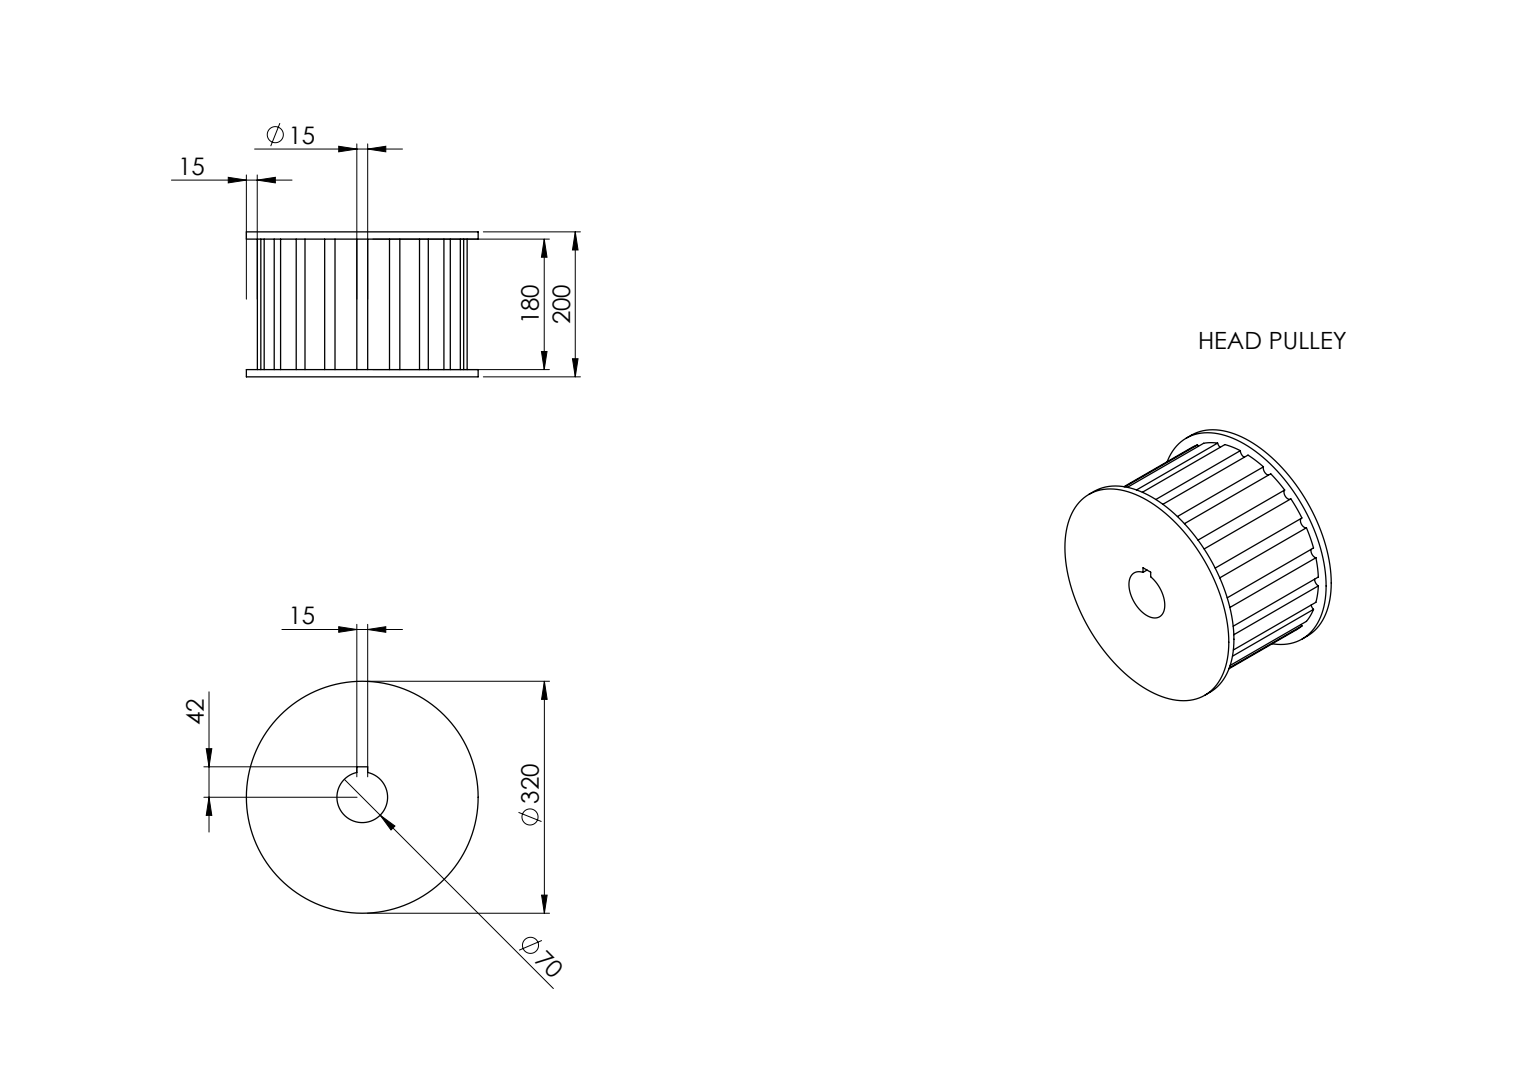
ISO-10303-21;
HEADER;
FILE_DESCRIPTION (('STEP AP214'),
    '1' );
FILE_NAME ('head pulley.step',
    '2026-10-31T03:46:07',
    ( '' ),
    ( '' ),
    'SwSTEP 2.0',
    'SolidWorks 2026',
    '' );
FILE_SCHEMA (( 'AUTOMOTIVE_DESIGN' ));
ENDSEC;

DATA;
#2=AXIS2_PLACEMENT_3D ( 'NONE', #6782, #12036, #15971 ) ;
#22=EDGE_CURVE ( 'NONE', #12572, #17693, #16078, .T. ) ;
#63=ORIENTED_EDGE ( 'NONE', *, *, #22259, .T. ) ;
#78=LINE ( 'NONE', #5499, #566 ) ;
#89=ORIENTED_EDGE ( 'NONE', *, *, #1676, .F. ) ;
#114=ORIENTED_EDGE ( 'NONE', *, *, #423, .T. ) ;
#116=EDGE_CURVE ( 'NONE', #3375, #7169, #11833, .T. ) ;
#119=DIRECTION ( 'NONE',  ( 1.000000000000000000, 0.000000000000000000, 0.000000000000000000 ) ) ;
#121=ORIENTED_EDGE ( 'NONE', *, *, #12195, .F. ) ;
#134=CARTESIAN_POINT ( 'NONE',  ( -91.18044947428953151, 112.7436279071528702, 90.00000000000000000 ) ) ;
#155=DIRECTION ( 'NONE',  ( -0.000000000000000000, 0.000000000000000000, 1.000000000000000000 ) ) ;
#158=EDGE_LOOP ( 'NONE', ( #17391, #12843, #343, #3950 ) ) ;
#213=CIRCLE ( 'NONE', #14875, 160.0000000000000000 ) ;
#217=CARTESIAN_POINT ( 'NONE',  ( 0.000000000000000000, 0.000000000000000000, 90.00000000000000000 ) ) ;
#229=DIRECTION ( 'NONE',  ( 0.000000000000000000, 0.000000000000000000, 1.000000000000000000 ) ) ;
#235=AXIS2_PLACEMENT_3D ( 'NONE', #16320, #23663, #13576 ) ;
#236=AXIS2_PLACEMENT_3D ( 'NONE', #4373, #19210, #636 ) ;
#258=LINE ( 'NONE', #11397, #17366 ) ;
#261=AXIS2_PLACEMENT_3D ( 'NONE', #2873, #10278, #8330 ) ;
#285=PRESENTATION_STYLE_ASSIGNMENT (( #3537 ) ) ;
#294=AXIS2_PLACEMENT_3D ( 'NONE', #882, #5000, #6440 ) ;
#298=LINE ( 'NONE', #3551, #3445 ) ;
#329=DIRECTION ( 'NONE',  ( 1.000000000000000000, 0.000000000000000000, 0.000000000000000000 ) ) ;
#333=AXIS2_PLACEMENT_3D ( 'NONE', #11581, #4410, #11450 ) ;
#343=ORIENTED_EDGE ( 'NONE', *, *, #12074, .F. ) ;
#369=VECTOR ( 'NONE', #13127, 1000.000000000000000 ) ;
#383=CARTESIAN_POINT ( 'NONE',  ( -144.8060344827586050, -7.497491405672223941, -2.775557561562891351E-14 ) ) ;
#395=CARTESIAN_POINT ( 'NONE',  ( 51.87806360044629628, 135.4018704341563364, -90.00000000000000000 ) ) ;
#399=CIRCLE ( 'NONE', #7721, 7.499999999999996447 ) ;
#402=EDGE_LOOP ( 'NONE', ( #16572, #22684, #22058, #9340 ) ) ;
#417=AXIS2_PLACEMENT_3D ( 'NONE', #10094, #19108, #10454 ) ;
#423=EDGE_CURVE ( 'NONE', #23301, #11044, #12932, .T. ) ;
#427=ADVANCED_FACE ( 'NONE', ( #15825 ), #831, .F. ) ;
#440=DIRECTION ( 'NONE',  ( 1.000000000000000000, 0.000000000000000000, 0.000000000000000000 ) ) ;
#450=ORIENTED_EDGE ( 'NONE', *, *, #16095, .T. ) ;
#452=CARTESIAN_POINT ( 'NONE',  ( 0.000000000000000000, 0.000000000000000000, 90.00000000000000000 ) ) ;
#461=EDGE_LOOP ( 'NONE', ( #908, #4370, #8639, #3777 ) ) ;
#466=DIRECTION ( 'NONE',  ( 0.000000000000000000, 0.000000000000000000, 1.000000000000000000 ) ) ;
#467=DIRECTION ( 'NONE',  ( 0.9510565162951580831, -0.3090169943749334069, 0.000000000000000000 ) ) ;
#501=EDGE_LOOP ( 'NONE', ( #8871, #21661, #12574, #4452 ) ) ;
#517=DIRECTION ( 'NONE',  ( -0.000000000000000000, -0.000000000000000000, 1.000000000000000000 ) ) ;
#519=ORIENTED_EDGE ( 'NONE', *, *, #14734, .F. ) ;
#533=ORIENTED_EDGE ( 'NONE', *, *, #2318, .F. ) ;
#536=FACE_OUTER_BOUND ( 'NONE', #16343, .T. ) ;
#548=DIRECTION ( 'NONE',  ( -3.700743415417187942E-15, 1.000000000000000000, 0.000000000000000000 ) ) ;
#554=CARTESIAN_POINT ( 'NONE',  ( 0.000000000000000000, 0.000000000000000000, -90.00000000000000000 ) ) ;
#566=VECTOR ( 'NONE', #11218, 1000.000000000000000 ) ;
#569=AXIS2_PLACEMENT_3D ( 'NONE', #10338, #15656, #17679 ) ;
#595=VECTOR ( 'NONE', #12133, 1000.000000000000000 ) ;
#599=ORIENTED_EDGE ( 'NONE', *, *, #1215, .T. ) ;
#601=VECTOR ( 'NONE', #6636, 1000.000000000000000 ) ;
#636=DIRECTION ( 'NONE',  ( 1.000000000000000000, 0.000000000000000000, 0.000000000000000000 ) ) ;
#649=CYLINDRICAL_SURFACE ( 'NONE', #1566, 160.0000000000000000 ) ;
#666=DIRECTION ( 'NONE',  ( -0.000000000000000000, -0.000000000000000000, 1.000000000000000000 ) ) ;
#669=CARTESIAN_POINT ( 'NONE',  ( 0.000000000000000000, 0.000000000000000000, -90.00000000000000000 ) ) ;
#680=ORIENTED_EDGE ( 'NONE', *, *, #10475, .T. ) ;
#701=CARTESIAN_POINT ( 'NONE',  ( 0.000000000000000000, 0.000000000000000000, -90.00000000000000000 ) ) ;
#724=LINE ( 'NONE', #11387, #3443 ) ;
#764=CIRCLE ( 'NONE', #10431, 7.500000000000000888 ) ;
#766=VERTEX_POINT ( 'NONE', #23002 ) ;
#772=ORIENTED_EDGE ( 'NONE', *, *, #4782, .T. ) ;
#796=DIRECTION ( 'NONE',  ( 0.000000000000000000, 0.000000000000000000, 1.000000000000000000 ) ) ;
#807=DIRECTION ( 'NONE',  ( 0.000000000000000000, -0.000000000000000000, 1.000000000000000000 ) ) ;
#811=CARTESIAN_POINT ( 'NONE',  ( 160.0000000000000000, 1.959434878635765210E-14, 100.0000000000000000 ) ) ;
#821=LINE ( 'NONE', #19284, #1182 ) ;
#831=CYLINDRICAL_SURFACE ( 'NONE', #5609, 7.500000000000007105 ) ;
#835=EDGE_CURVE ( 'NONE', #2765, #10209, #1509, .T. ) ;
#856=CARTESIAN_POINT ( 'NONE',  ( 37.61698748598423947, 140.0355749532214702, -90.00000000000000000 ) ) ;
#857=ORIENTED_EDGE ( 'NONE', *, *, #7014, .T. ) ;
#880=VERTEX_POINT ( 'NONE', #13468 ) ;
#882=CARTESIAN_POINT ( 'NONE',  ( -44.80746418436648071, -137.9031948627975908, -90.00000000000000000 ) ) ;
#884=LINE ( 'NONE', #23340, #6165 ) ;
#895=VECTOR ( 'NONE', #10102, 1000.000000000000000 ) ;
#906=CYLINDRICAL_SURFACE ( 'NONE', #17761, 145.0000000000000284 ) ;
#908=ORIENTED_EDGE ( 'NONE', *, *, #12705, .F. ) ;
#909=DIRECTION ( 'NONE',  ( 0.000000000000000000, 0.000000000000000000, 1.000000000000000000 ) ) ;
#915=CIRCLE ( 'NONE', #6313, 7.500000000000001776 ) ;
#921=CARTESIAN_POINT ( 'NONE',  ( 7.497491405671719455, 144.8060344827586334, 90.00000000000000000 ) ) ;
#923=ORIENTED_EDGE ( 'NONE', *, *, #16478, .F. ) ;
#947=LINE ( 'NONE', #17750, #601 ) ;
#952=AXIS2_PLACEMENT_3D ( 'NONE', #10071, #9939, #18964 ) ;
#976=CARTESIAN_POINT ( 'NONE',  ( 0.000000000000000000, 0.000000000000000000, -90.00000000000000000 ) ) ;
#991=EDGE_CURVE ( 'NONE', #20344, #17672, #1333, .T. ) ;
#1001=FACE_OUTER_BOUND ( 'NONE', #4174, .T. ) ;
#1004=DIRECTION ( 'NONE',  ( 1.000000000000000000, 0.000000000000000000, 0.000000000000000000 ) ) ;
#1009=DIRECTION ( 'NONE',  ( 0.000000000000000000, 0.000000000000000000, 1.000000000000000000 ) ) ;
#1016=DIRECTION ( 'NONE',  ( -0.000000000000000000, -0.000000000000000000, 1.000000000000000000 ) ) ;
#1032=DIRECTION ( 'NONE',  ( -0.000000000000000000, -0.000000000000000000, 1.000000000000000000 ) ) ;
#1040=CARTESIAN_POINT ( 'NONE',  ( 0.000000000000000000, 0.000000000000000000, -90.00000000000000000 ) ) ;
#1047=DIRECTION ( 'NONE',  ( 1.000000000000000000, 0.000000000000000000, 0.000000000000000000 ) ) ;
#1053=CYLINDRICAL_SURFACE ( 'NONE', #6841, 145.0000000000000284 ) ;
#1067=CYLINDRICAL_SURFACE ( 'NONE', #22936, 145.0000000000000284 ) ;
#1083=VECTOR ( 'NONE', #9378, 1000.000000000000000 ) ;
#1085=ORIENTED_EDGE ( 'NONE', *, *, #2157, .T. ) ;
#1091=CARTESIAN_POINT ( 'NONE',  ( -44.80746418436748968, 137.9031948627972781, 90.00000000000000000 ) ) ;
#1131=VERTEX_POINT ( 'NONE', #6538 ) ;
#1141=CARTESIAN_POINT ( 'NONE',  ( 144.8060344827585482, 7.497491405673236464, -90.00000000000000000 ) ) ;
#1148=VECTOR ( 'NONE', #21385, 1000.000000000000000 ) ;
#1149=DIRECTION ( 'NONE',  ( -0.000000000000000000, -0.000000000000000000, 1.000000000000000000 ) ) ;
#1154=DIRECTION ( 'NONE',  ( 1.000000000000000000, 0.000000000000000000, 0.000000000000000000 ) ) ;
#1165=AXIS2_PLACEMENT_3D ( 'NONE', #13877, #15664, #1154 ) ;
#1182=VECTOR ( 'NONE', #15686, 1000.000000000000000 ) ;
#1215=EDGE_CURVE ( 'NONE', #10931, #3015, #16546, .T. ) ;
#1229=CARTESIAN_POINT ( 'NONE',  ( 117.3074641843682144, -85.22886158240748955, -90.00000000000000000 ) ) ;
#1243=ORIENTED_EDGE ( 'NONE', *, *, #1911, .T. ) ;
#1244=EDGE_CURVE ( 'NONE', #12407, #10771, #17975, .T. ) ;
#1251=ORIENTED_EDGE ( 'NONE', *, *, #2208, .F. ) ;
#1256=CARTESIAN_POINT ( 'NONE',  ( 0.000000000000000000, 0.000000000000000000, -90.00000000000000000 ) ) ;
#1259=FACE_OUTER_BOUND ( 'NONE', #10230, .T. ) ;
#1263=FACE_OUTER_BOUND ( 'NONE', #6850, .T. ) ;
#1267=CARTESIAN_POINT ( 'NONE',  ( 0.000000000000000000, 0.000000000000000000, -90.00000000000000000 ) ) ;
#1278=CARTESIAN_POINT ( 'NONE',  ( 0.000000000000000000, 0.000000000000000000, -90.00000000000000000 ) ) ;
#1295=VERTEX_POINT ( 'NONE', #11268 ) ;
#1300=ADVANCED_FACE ( 'NONE', ( #18575 ), #14405, .F. ) ;
#1307=EDGE_CURVE ( 'NONE', #12981, #9371, #16811, .T. ) ;
#1312=DIRECTION ( 'NONE',  ( 0.000000000000000000, 0.000000000000000000, 1.000000000000000000 ) ) ;
#1316=CARTESIAN_POINT ( 'NONE',  ( -91.18044947428876412, -112.7436279071535239, -90.00000000000000000 ) ) ;
#1317=CIRCLE ( 'NONE', #7476, 7.499999999999996447 ) ;
#1322=VERTEX_POINT ( 'NONE', #17268 ) ;
#1323=DIRECTION ( 'NONE',  ( -0.000000000000000000, -0.000000000000000000, 1.000000000000000000 ) ) ;
#1333=CIRCLE ( 'NONE', #952, 145.0000000000000284 ) ;
#1368=CARTESIAN_POINT ( 'NONE',  ( -44.80746418436648071, -137.9031948627975908, -90.00000000000000000 ) ) ;
#1389=DIRECTION ( 'NONE',  ( 0.5877852522924826850, -0.8090169943749405679, 0.000000000000000000 ) ) ;
#1402=ORIENTED_EDGE ( 'NONE', *, *, #2339, .F. ) ;
#1406=FACE_OUTER_BOUND ( 'NONE', #5182, .T. ) ;
#1444=AXIS2_PLACEMENT_3D ( 'NONE', #23645, #5648, #23539 ) ;
#1456=CIRCLE ( 'NONE', #13459, 160.0000000000000000 ) ;
#1462=CARTESIAN_POINT ( 'NONE',  ( 0.000000000000000000, 0.000000000000000000, 100.0000000000000000 ) ) ;
#1480=ORIENTED_EDGE ( 'NONE', *, *, #116, .F. ) ;
#1486=ORIENTED_EDGE ( 'NONE', *, *, #8980, .T. ) ;
#1492=PRODUCT_DEFINITION_SHAPE ( 'NONE', 'NONE',  #21557 ) ;
#1498=AXIS2_PLACEMENT_3D ( 'NONE', #10621, #14371, #12334 ) ;
#1509=LINE ( 'NONE', #3191, #4429 ) ;
#1513=CIRCLE ( 'NONE', #7691, 7.500000000000001776 ) ;
#1514=CARTESIAN_POINT ( 'NONE',  ( 85.22886158240706322, 117.3074641843685129, -90.00000000000000000 ) ) ;
#1518=CIRCLE ( 'NONE', #16954, 7.499999999999998224 ) ;
#1533=DIRECTION ( 'NONE',  ( 0.000000000000000000, 0.000000000000000000, 1.000000000000000000 ) ) ;
#1541=DIRECTION ( 'NONE',  ( 0.000000000000000000, -0.000000000000000000, 1.000000000000000000 ) ) ;
#1565=CIRCLE ( 'NONE', #6182, 7.500000000000000888 ) ;
#1566=AXIS2_PLACEMENT_3D ( 'NONE', #2201, #7778, #5721 ) ;
#1570=DIRECTION ( 'NONE',  ( 1.000000000000000000, 0.000000000000000000, 0.000000000000000000 ) ) ;
#1571=ORIENTED_EDGE ( 'NONE', *, *, #18407, .T. ) ;
#1577=FACE_OUTER_BOUND ( 'NONE', #7495, .T. ) ;
#1579=DIRECTION ( 'NONE',  ( -0.000000000000000000, -0.000000000000000000, -1.000000000000000000 ) ) ;
#1582=ORIENTED_EDGE ( 'NONE', *, *, #991, .T. ) ;
#1595=CARTESIAN_POINT ( 'NONE',  ( -137.9031948627971076, -44.80746418436799416, -90.00000000000000000 ) ) ;
#1604=CARTESIAN_POINT ( 'NONE',  ( 0.000000000000000000, 0.000000000000000000, 90.00000000000000000 ) ) ;
#1629=PLANE ( 'NONE',  #11213 ) ;
#1634=DIRECTION ( 'NONE',  ( 0.3090169943749589421, -0.9510565162951498674, 0.000000000000000000 ) ) ;
#1676=EDGE_CURVE ( 'NONE', #18305, #13461, #5588, .T. ) ;
#1696=DIRECTION ( 'NONE',  ( -0.000000000000000000, -0.000000000000000000, -1.000000000000000000 ) ) ;
#1737=DIRECTION ( 'NONE',  ( 0.000000000000000000, -0.000000000000000000, 1.000000000000000000 ) ) ;
#1741=CARTESIAN_POINT ( 'NONE',  ( 145.0000000000000284, 1.518794382396763073E-12, -90.00000000000000000 ) ) ;
#1747=DIRECTION ( 'NONE',  ( 0.000000000000000000, 0.000000000000000000, 1.000000000000000000 ) ) ;
#1762=EDGE_CURVE ( 'NONE', #13072, #14205, #10366, .T. ) ;
#1784=CARTESIAN_POINT ( 'NONE',  ( 0.000000000000000000, 0.000000000000000000, -90.00000000000000000 ) ) ;
#1791=DIRECTION ( 'NONE',  ( 0.000000000000000000, -0.000000000000000000, 1.000000000000000000 ) ) ;
#1794=AXIS2_PLACEMENT_3D ( 'NONE', #14987, #11136, #18938 ) ;
#1827=CARTESIAN_POINT ( 'NONE',  ( -135.4018704341557680, 51.87806360044768184, -2.775557561562891351E-14 ) ) ;
#1876=DIRECTION ( 'NONE',  ( 0.8090169943749468962, 0.5877852522924740253, 0.000000000000000000 ) ) ;
#1883=AXIS2_PLACEMENT_3D ( 'NONE', #17096, #15181, #18896 ) ;
#1892=CARTESIAN_POINT ( 'NONE',  ( -121.5574576620394112, -79.04925354955290118, 90.00000000000000000 ) ) ;
#1908=CARTESIAN_POINT ( 'NONE',  ( -137.9031948627974486, 44.80746418436699940, -90.00000000000000000 ) ) ;
#1910=CIRCLE ( 'NONE', #9647, 7.499999999999998224 ) ;
#1911=EDGE_CURVE ( 'NONE', #17693, #2497, #16893, .T. ) ;
#1951=EDGE_CURVE ( 'NONE', #20344, #18305, #14697, .T. ) ;
#1977=ADVANCED_FACE ( 'NONE', ( #5259 ), #11076, .F. ) ;
#1997=DIRECTION ( 'NONE',  ( 0.000000000000000000, 0.000000000000000000, 1.000000000000000000 ) ) ;
#2001=AXIS2_PLACEMENT_3D ( 'NONE', #14523, #21858, #3611 ) ;
#2013=CARTESIAN_POINT ( 'NONE',  ( -77.72886158240795851, -117.3074641843678876, 90.00000000000000000 ) ) ;
#2032=EDGE_CURVE ( 'NONE', #17746, #2765, #11464, .T. ) ;
#2033=EDGE_CURVE ( 'NONE', #11764, #2480, #23769, .T. ) ;
#2046=CYLINDRICAL_SURFACE ( 'NONE', #9224, 145.0000000000000284 ) ;
#2077=CARTESIAN_POINT ( 'NONE',  ( -160.0000000000000000, 0.000000000000000000, 100.0000000000000000 ) ) ;
#2080=CARTESIAN_POINT ( 'NONE',  ( 112.7436279071538792, -91.18044947428829516, 90.00000000000000000 ) ) ;
#2081=ORIENTED_EDGE ( 'NONE', *, *, #10315, .T. ) ;
#2083=( LENGTH_UNIT ( ) NAMED_UNIT ( * ) SI_UNIT ( .MILLI., .METRE. ) );
#2090=DIRECTION ( 'NONE',  ( 0.000000000000000000, 0.000000000000000000, -1.000000000000000000 ) ) ;
#2094=CARTESIAN_POINT ( 'NONE',  ( 135.4018704341550290, 51.87806360044960030, -2.775557561562891351E-14 ) ) ;
#2121=DIRECTION ( 'NONE',  ( 0.000000000000000000, 0.000000000000000000, 1.000000000000000000 ) ) ;
#2129=PLANE ( 'NONE',  #2515 ) ;
#2155=ORIENTED_EDGE ( 'NONE', *, *, #11016, .F. ) ;
#2157=EDGE_CURVE ( 'NONE', #11764, #22779, #3251, .T. ) ;
#2159=AXIS2_PLACEMENT_3D ( 'NONE', #16619, #18062, #16480 ) ;
#2164=DIRECTION ( 'NONE',  ( -0.8090169943749507819, 0.5877852522924686962, 0.000000000000000000 ) ) ;
#2165=DIRECTION ( 'NONE',  ( 1.000000000000000000, 0.000000000000000000, 0.000000000000000000 ) ) ;
#2185=ORIENTED_EDGE ( 'NONE', *, *, #4517, .F. ) ;
#2187=CYLINDRICAL_SURFACE ( 'NONE', #236, 7.500000000000007105 ) ;
#2191=PLANE ( 'NONE',  #14998 ) ;
#2201=CARTESIAN_POINT ( 'NONE',  ( 0.000000000000000000, 0.000000000000000000, 100.0000000000000000 ) ) ;
#2202=AXIS2_PLACEMENT_3D ( 'NONE', #14375, #18086, #9030 ) ;
#2208=EDGE_CURVE ( 'NONE', #17463, #13673, #4416, .T. ) ;
#2230=VECTOR ( 'NONE', #5125, 1000.000000000000000 ) ;
#2239=DIRECTION ( 'NONE',  ( 0.000000000000000000, 0.000000000000000000, 1.000000000000000000 ) ) ;
#2252=DIRECTION ( 'NONE',  ( 0.000000000000000000, 0.000000000000000000, 1.000000000000000000 ) ) ;
#2258=PLANE ( 'NONE',  #4571 ) ;
#2283=AXIS2_PLACEMENT_3D ( 'NONE', #6230, #5097, #15543 ) ;
#2285=CIRCLE ( 'NONE', #16192, 145.0000000000000284 ) ;
#2292=VECTOR ( 'NONE', #4806, 1000.000000000000000 ) ;
#2303=ORIENTED_EDGE ( 'NONE', *, *, #4569, .F. ) ;
#2314=FACE_OUTER_BOUND ( 'NONE', #10322, .T. ) ;
#2317=CYLINDRICAL_SURFACE ( 'NONE', #4211, 145.0000000000000284 ) ;
#2318=EDGE_CURVE ( 'NONE', #16501, #13664, #5742, .T. ) ;
#2320=VERTEX_POINT ( 'NONE', #10099 ) ;
#2339=EDGE_CURVE ( 'NONE', #6206, #13931, #4971, .T. ) ;
#2351=DIRECTION ( 'NONE',  ( -0.000000000000000000, 0.000000000000000000, 1.000000000000000000 ) ) ;
#2361=CARTESIAN_POINT ( 'NONE',  ( 160.0000000000000000, 1.959434878635765210E-14, 100.0000000000000000 ) ) ;
#2370=CARTESIAN_POINT ( 'NONE',  ( 0.000000000000000000, 0.000000000000000000, 90.00000000000000000 ) ) ;
#2376=EDGE_CURVE ( 'NONE', #18600, #18149, #23477, .T. ) ;
#2406=ORIENTED_EDGE ( 'NONE', *, *, #20105, .T. ) ;
#2441=DIRECTION ( 'NONE',  ( 1.000000000000000000, 0.000000000000000000, 0.000000000000000000 ) ) ;
#2459=ORIENTED_EDGE ( 'NONE', *, *, #4998, .T. ) ;
#2461=CARTESIAN_POINT ( 'NONE',  ( 140.0355749532213281, -37.61698748598472264, 90.00000000000000000 ) ) ;
#2475=DIRECTION ( 'NONE',  ( 0.000000000000000000, 0.000000000000000000, 1.000000000000000000 ) ) ;
#2480=VERTEX_POINT ( 'NONE', #5349 ) ;
#2483=LINE ( 'NONE', #20962, #9282 ) ;
#2497=VERTEX_POINT ( 'NONE', #8874 ) ;
#2509=ORIENTED_EDGE ( 'NONE', *, *, #11719, .T. ) ;
#2515=AXIS2_PLACEMENT_3D ( 'NONE', #3941, #7574, #9521 ) ;
#2575=EDGE_CURVE ( 'NONE', #3378, #2646, #3889, .T. ) ;
#2579=ORIENTED_EDGE ( 'NONE', *, *, #13734, .F. ) ;
#2601=EDGE_CURVE ( 'NONE', #1295, #18149, #20390, .T. ) ;
#2612=EDGE_LOOP ( 'NONE', ( #8421, #21186, #22709, #21255 ) ) ;
#2636=EDGE_CURVE ( 'NONE', #21483, #4937, #16940, .T. ) ;
#2644=LINE ( 'NONE', #6511, #4380 ) ;
#2645=ORIENTED_EDGE ( 'NONE', *, *, #6630, .T. ) ;
#2646=VERTEX_POINT ( 'NONE', #16812 ) ;
#2653=AXIS2_PLACEMENT_3D ( 'NONE', #18912, #22648, #19018 ) ;
#2663=ADVANCED_FACE ( 'NONE', ( #5831 ), #2317, .T. ) ;
#2667=CARTESIAN_POINT ( 'NONE',  ( -37.61698748598514896, -140.0355749532212428, -2.775557561562891351E-14 ) ) ;
#2670=AXIS2_PLACEMENT_3D ( 'NONE', #17531, #19703, #21287 ) ;
#2676=CARTESIAN_POINT ( 'NONE',  ( -51.87806360044817922, 135.4018704341556258, -2.775557561562891351E-14 ) ) ;
#2684=ORIENTED_EDGE ( 'NONE', *, *, #6466, .F. ) ;
#2710=DIRECTION ( 'NONE',  ( 0.3090169943749441761, 0.9510565162951546414, 0.000000000000000000 ) ) ;
#2716=LINE ( 'NONE', #21061, #895 ) ;
#2720=ORIENTED_EDGE ( 'NONE', *, *, #16990, .F. ) ;
#2745=DIRECTION ( 'NONE',  ( 1.000000000000000000, 0.000000000000000000, 0.000000000000000000 ) ) ;
#2747=DIRECTION ( 'NONE',  ( -0.000000000000000000, 0.000000000000000000, 1.000000000000000000 ) ) ;
#2760=EDGE_LOOP ( 'NONE', ( #18334, #15913 ) ) ;
#2765=VERTEX_POINT ( 'NONE', #15377 ) ;
#2777=EDGE_CURVE ( 'NONE', #9321, #21395, #16651, .T. ) ;
#2803=LINE ( 'NONE', #15632, #15852 ) ;
#2826=CARTESIAN_POINT ( 'NONE',  ( -44.80746418436648071, -137.9031948627975908, 90.00000000000000000 ) ) ;
#2829=DIRECTION ( 'NONE',  ( 0.000000000000000000, 0.000000000000000000, 1.000000000000000000 ) ) ;
#2831=DIRECTION ( 'NONE',  ( 1.000000000000000000, 0.000000000000000000, 0.000000000000000000 ) ) ;
#2844=ORIENTED_EDGE ( 'NONE', *, *, #19085, .F. ) ;
#2852=CARTESIAN_POINT ( 'NONE',  ( -112.7436279071531828, 91.18044947428913360, -90.00000000000000000 ) ) ;
#2854=AXIS2_PLACEMENT_3D ( 'NONE', #16273, #21451, #1634 ) ;
#2873=CARTESIAN_POINT ( 'NONE',  ( 0.000000000000000000, 0.000000000000000000, -90.00000000000000000 ) ) ;
#2874=AXIS2_PLACEMENT_3D ( 'NONE', #20053, #18347, #8961 ) ;
#2877=CARTESIAN_POINT ( 'NONE',  ( 79.04925354955072692, 121.5574576620408322, 90.00000000000000000 ) ) ;
#2884=CIRCLE ( 'NONE', #9085, 145.0000000000000284 ) ;
#2912=CIRCLE ( 'NONE', #18734, 145.0000000000000284 ) ;
#2914=DIRECTION ( 'NONE',  ( 0.000000000000000000, 0.000000000000000000, -1.000000000000000000 ) ) ;
#2919=ORIENTED_EDGE ( 'NONE', *, *, #13068, .T. ) ;
#2944=EDGE_CURVE ( 'NONE', #15856, #9608, #22362, .T. ) ;
#2947=ORIENTED_EDGE ( 'NONE', *, *, #20986, .F. ) ;
#2957=CARTESIAN_POINT ( 'NONE',  ( 85.22886158240964960, -117.3074641843666370, 90.00000000000000000 ) ) ;
#2990=DIRECTION ( 'NONE',  ( 1.000000000000000000, 0.000000000000000000, 0.000000000000000000 ) ) ;
#3015=VERTEX_POINT ( 'NONE', #10497 ) ;
#3031=EDGE_CURVE ( 'NONE', #21305, #6640, #16542, .T. ) ;
#3070=CARTESIAN_POINT ( 'NONE',  ( -7.497491405671719455, 144.8060344827586334, -2.775557561562891351E-14 ) ) ;
#3075=EDGE_LOOP ( 'NONE', ( #16565, #17357, #19371, #4735, #9836, #18694 ) ) ;
#3108=AXIS2_PLACEMENT_3D ( 'NONE', #16381, #1747, #18295 ) ;
#3110=VERTEX_POINT ( 'NONE', #6364 ) ;
#3130=CARTESIAN_POINT ( 'NONE',  ( 112.7436279071518612, 91.18044947429076785, 90.00000000000000000 ) ) ;
#3142=VERTEX_POINT ( 'NONE', #921 ) ;
#3152=DIRECTION ( 'NONE',  ( 1.000000000000000000, 0.000000000000000000, 0.000000000000000000 ) ) ;
#3182=CARTESIAN_POINT ( 'NONE',  ( -112.7436279071525433, -91.18044947428992941, 90.00000000000000000 ) ) ;
#3185=ORIENTED_EDGE ( 'NONE', *, *, #10970, .T. ) ;
#3187=ORIENTED_EDGE ( 'NONE', *, *, #3737, .F. ) ;
#3191=CARTESIAN_POINT ( 'NONE',  ( -37.61698748598617925, 140.0355749532209870, -2.775557561562891351E-14 ) ) ;
#3207=DIRECTION ( 'NONE',  ( -0.000000000000000000, -0.000000000000000000, 1.000000000000000000 ) ) ;
#3239=DIRECTION ( 'NONE',  ( 0.000000000000000000, 0.000000000000000000, 1.000000000000000000 ) ) ;
#3241=EDGE_CURVE ( 'NONE', #5473, #13502, #5147, .T. ) ;
#3251=CIRCLE ( 'NONE', #22915, 7.500000000000004441 ) ;
#3258=CIRCLE ( 'NONE', #9468, 160.0000000000000000 ) ;
#3267=DIRECTION ( 'NONE',  ( 0.000000000000000000, -0.000000000000000000, 1.000000000000000000 ) ) ;
#3291=AXIS2_PLACEMENT_3D ( 'NONE', #1256, #10212, #10333 ) ;
#3299=CARTESIAN_POINT ( 'NONE',  ( -79.04925354955163641, -121.5574576620402496, -90.00000000000000000 ) ) ;
#3305=EDGE_CURVE ( 'NONE', #12407, #18161, #19576, .T. ) ;
#3326=DIRECTION ( 'NONE',  ( 1.000000000000000000, 0.000000000000000000, 0.000000000000000000 ) ) ;
#3331=ADVANCED_FACE ( 'NONE', ( #6798 ), #8503, .F. ) ;
#3350=VECTOR ( 'NONE', #14502, 1000.000000000000000 ) ;
#3360=CARTESIAN_POINT ( 'NONE',  ( 0.000000000000000000, 0.000000000000000000, 100.0000000000000000 ) ) ;
#3370=CARTESIAN_POINT ( 'NONE',  ( 85.22886158240964960, -117.3074641843666370, -90.00000000000000000 ) ) ;
#3375=VERTEX_POINT ( 'NONE', #13973 ) ;
#3378=VERTEX_POINT ( 'NONE', #12156 ) ;
#3380=VECTOR ( 'NONE', #3868, 1000.000000000000000 ) ;
#3385=AXIS2_PLACEMENT_3D ( 'NONE', #22286, #16863, #17233 ) ;
#3401=VECTOR ( 'NONE', #9352, 1000.000000000000000 ) ;
#3407=CARTESIAN_POINT ( 'NONE',  ( 0.000000000000000000, 0.000000000000000000, -90.00000000000000000 ) ) ;
#3421=VECTOR ( 'NONE', #4763, 1000.000000000000000 ) ;
#3429=ORIENTED_EDGE ( 'NONE', *, *, #21555, .F. ) ;
#3443=VECTOR ( 'NONE', #13694, 1000.000000000000000 ) ;
#3445=VECTOR ( 'NONE', #1737, 1000.000000000000000 ) ;
#3446=VECTOR ( 'NONE', #13913, 1000.000000000000000 ) ;
#3471=CARTESIAN_POINT ( 'NONE',  ( 0.000000000000000000, 0.000000000000000000, -100.0000000000000000 ) ) ;
#3475=VECTOR ( 'NONE', #2914, 1000.000000000000000 ) ;
#3483=CARTESIAN_POINT ( 'NONE',  ( -85.22886158240879695, 117.3074641843673049, -90.00000000000000000 ) ) ;
#3489=AXIS2_PLACEMENT_3D ( 'NONE', #13729, #22848, #11795 ) ;
#3497=DIRECTION ( 'NONE',  ( 1.000000000000000000, 0.000000000000000000, 0.000000000000000000 ) ) ;
#3517=ORIENTED_EDGE ( 'NONE', *, *, #16077, .T. ) ;
#3524=ORIENTED_EDGE ( 'NONE', *, *, #13067, .F. ) ;
#3537=SURFACE_STYLE_USAGE ( .BOTH. , #16715 ) ;
#3543=CARTESIAN_POINT ( 'NONE',  ( 0.000000000000000000, 0.000000000000000000, -90.00000000000000000 ) ) ;
#3545=EDGE_CURVE ( 'NONE', #7634, #10526, #9256, .T. ) ;
#3551=CARTESIAN_POINT ( 'NONE',  ( -79.04925354955163641, -121.5574576620402496, -2.775557561562891351E-14 ) ) ;
#3587=ORIENTED_EDGE ( 'NONE', *, *, #6215, .T. ) ;
#3611=DIRECTION ( 'NONE',  ( 0.3090169943749441761, 0.9510565162951546414, 0.000000000000000000 ) ) ;
#3633=EDGE_CURVE ( 'NONE', #13320, #22438, #298, .T. ) ;
#3650=DIRECTION ( 'NONE',  ( 1.000000000000000000, 0.000000000000000000, 0.000000000000000000 ) ) ;
#3670=CARTESIAN_POINT ( 'NONE',  ( 112.7436279071538792, -91.18044947428829516, -90.00000000000000000 ) ) ;
#3685=CARTESIAN_POINT ( 'NONE',  ( 0.000000000000000000, 0.000000000000000000, 90.00000000000000000 ) ) ;
#3693=VERTEX_POINT ( 'NONE', #15407 ) ;
#3694=EDGE_CURVE ( 'NONE', #12407, #19135, #4150, .T. ) ;
#3723=DIRECTION ( 'NONE',  ( 0.000000000000000000, 0.000000000000000000, 1.000000000000000000 ) ) ;
#3735=LINE ( 'NONE', #16913, #3380 ) ;
#3737=EDGE_CURVE ( 'NONE', #19135, #13502, #884, .T. ) ;
#3755=CIRCLE ( 'NONE', #17284, 7.499999999999998224 ) ;
#3769=DIRECTION ( 'NONE',  ( 1.000000000000000000, 0.000000000000000000, 0.000000000000000000 ) ) ;
#3777=ORIENTED_EDGE ( 'NONE', *, *, #8405, .F. ) ;
#3796=CARTESIAN_POINT ( 'NONE',  ( 135.4018704341561374, -51.87806360044677945, -2.775557561562891351E-14 ) ) ;
#3828=EDGE_LOOP ( 'NONE', ( #13650, #12892, #17242, #8630 ) ) ;
#3849=EDGE_CURVE ( 'NONE', #9726, #1322, #23504, .T. ) ;
#3859=AXIS2_PLACEMENT_3D ( 'NONE', #14257, #5168, #17735 ) ;
#3868=DIRECTION ( 'NONE',  ( 0.000000000000000000, -0.000000000000000000, 1.000000000000000000 ) ) ;
#3877=ORIENTED_EDGE ( 'NONE', *, *, #18176, .T. ) ;
#3883=EDGE_CURVE ( 'NONE', #22438, #17622, #9242, .T. ) ;
#3889=LINE ( 'NONE', #1827, #19244 ) ;
#3897=LINE ( 'NONE', #20550, #18071 ) ;
#3906=DIRECTION ( 'NONE',  ( 1.000000000000000000, 0.000000000000000000, 0.000000000000000000 ) ) ;
#3912=DIRECTION ( 'NONE',  ( 0.000000000000000000, 0.000000000000000000, 1.000000000000000000 ) ) ;
#3941=CARTESIAN_POINT ( 'NONE',  ( 7.499999999999999112, 0.000000000000000000, -100.0000000000000000 ) ) ;
#3950=ORIENTED_EDGE ( 'NONE', *, *, #21410, .F. ) ;
#3958=EDGE_LOOP ( 'NONE', ( #23510, #8785, #8693, #9032 ) ) ;
#3974=CARTESIAN_POINT ( 'NONE',  ( -85.22886158240795851, -117.3074641843678876, -90.00000000000000000 ) ) ;
#3976=DIRECTION ( 'NONE',  ( -0.000000000000000000, -0.000000000000000000, 1.000000000000000000 ) ) ;
#3988=AXIS2_PLACEMENT_3D ( 'NONE', #15544, #17350, #4660 ) ;
#4000=LINE ( 'NONE', #13608, #10803 ) ;
#4001=FACE_OUTER_BOUND ( 'NONE', #12359, .T. ) ;
#4031=CARTESIAN_POINT ( 'NONE',  ( -77.72886158240878274, 117.3074641843673049, -90.00000000000000000 ) ) ;
#4048=CYLINDRICAL_SURFACE ( 'NONE', #2653, 160.0000000000000000 ) ;
#4075=ADVANCED_FACE ( 'NONE', ( #8134 ), #22476, .F. ) ;
#4109=EDGE_CURVE ( 'NONE', #11121, #15263, #8595, .T. ) ;
#4114=VERTEX_POINT ( 'NONE', #14301 ) ;
#4115=ADVANCED_FACE ( 'NONE', ( #8484 ), #21150, .F. ) ;
#4119=ORIENTED_EDGE ( 'NONE', *, *, #15493, .F. ) ;
#4126=DIRECTION ( 'NONE',  ( -0.000000000000000000, -0.000000000000000000, 1.000000000000000000 ) ) ;
#4150=LINE ( 'NONE', #22390, #4613 ) ;
#4165=DIRECTION ( 'NONE',  ( -0.000000000000000000, -0.000000000000000000, 1.000000000000000000 ) ) ;
#4166=AXIS2_PLACEMENT_3D ( 'NONE', #1514, #18396, #9255 ) ;
#4174=EDGE_LOOP ( 'NONE', ( #13858, #6378, #10101, #1243 ) ) ;
#4177=DIRECTION ( 'NONE',  ( 0.000000000000000000, 0.000000000000000000, 1.000000000000000000 ) ) ;
#4185=FACE_OUTER_BOUND ( 'NONE', #13720, .T. ) ;
#4197=CARTESIAN_POINT ( 'NONE',  ( -35.00000000000000711, 4.286263797015737285E-15, -100.0000000000000000 ) ) ;
#4204=CIRCLE ( 'NONE', #18115, 145.0000000000000284 ) ;
#4211=AXIS2_PLACEMENT_3D ( 'NONE', #11177, #18722, #15143 ) ;
#4229=CARTESIAN_POINT ( 'NONE',  ( 160.0000000000000000, 1.959434878635765210E-14, -90.00000000000000000 ) ) ;
#4248=ORIENTED_EDGE ( 'NONE', *, *, #3545, .F. ) ;
#4258=DIRECTION ( 'NONE',  ( 1.000000000000000000, 0.000000000000000000, 0.000000000000000000 ) ) ;
#4260=ORIENTED_EDGE ( 'NONE', *, *, #22259, .F. ) ;
#4262=ADVANCED_FACE ( 'NONE', ( #10789 ), #16213, .F. ) ;
#4268=VERTEX_POINT ( 'NONE', #16553 ) ;
#4275=DIRECTION ( 'NONE',  ( -0.000000000000000000, -0.000000000000000000, 1.000000000000000000 ) ) ;
#4280=CARTESIAN_POINT ( 'NONE',  ( 0.000000000000000000, 145.0000000000000284, -90.00000000000000000 ) ) ;
#4287=ORIENTED_EDGE ( 'NONE', *, *, #12558, .F. ) ;
#4290=ORIENTED_EDGE ( 'NONE', *, *, #2376, .T. ) ;
#4310=LINE ( 'NONE', #6244, #6893 ) ;
#4327=DIRECTION ( 'NONE',  ( 0.000000000000000000, 0.000000000000000000, 1.000000000000000000 ) ) ;
#4338=DIRECTION ( 'NONE',  ( -0.000000000000000000, -0.000000000000000000, 1.000000000000000000 ) ) ;
#4365=DIRECTION ( 'NONE',  ( -0.000000000000000000, -0.000000000000000000, -1.000000000000000000 ) ) ;
#4370=ORIENTED_EDGE ( 'NONE', *, *, #8154, .T. ) ;
#4373=CARTESIAN_POINT ( 'NONE',  ( -145.0000000000000284, -5.062647941322544249E-13, -90.00000000000000000 ) ) ;
#4380=VECTOR ( 'NONE', #17614, 1000.000000000000000 ) ;
#4389=CARTESIAN_POINT ( 'NONE',  ( 35.00000000000000711, 0.000000000000000000, -100.0000000000000000 ) ) ;
#4404=ORIENTED_EDGE ( 'NONE', *, *, #6169, .T. ) ;
#4410=DIRECTION ( 'NONE',  ( 0.000000000000000000, 0.000000000000000000, 1.000000000000000000 ) ) ;
#4416=CIRCLE ( 'NONE', #13715, 7.500000000000000000 ) ;
#4427=AXIS2_PLACEMENT_3D ( 'NONE', #17887, #21386, #11899 ) ;
#4429=VECTOR ( 'NONE', #12549, 1000.000000000000000 ) ;
#4432=EDGE_CURVE ( 'NONE', #10931, #5086, #3258, .T. ) ;
#4452=ORIENTED_EDGE ( 'NONE', *, *, #13396, .F. ) ;
#4486=VECTOR ( 'NONE', #2090, 1000.000000000000000 ) ;
#4488=CARTESIAN_POINT ( 'NONE',  ( 0.000000000000000000, 0.000000000000000000, 90.00000000000000000 ) ) ;
#4489=ORIENTED_EDGE ( 'NONE', *, *, #17444, .T. ) ;
#4490=EDGE_CURVE ( 'NONE', #766, #5818, #11806, .T. ) ;
#4514=DIRECTION ( 'NONE',  ( -0.000000000000000000, 1.000000000000000000, 0.000000000000000000 ) ) ;
#4516=VERTEX_POINT ( 'NONE', #12114 ) ;
#4517=EDGE_CURVE ( 'NONE', #22779, #17746, #947, .T. ) ;
#4521=CYLINDRICAL_SURFACE ( 'NONE', #15666, 7.500000000000007105 ) ;
#4522=ORIENTED_EDGE ( 'NONE', *, *, #8740, .T. ) ;
#4527=DIRECTION ( 'NONE',  ( -0.9510565162951557516, 0.3090169943749406234, 0.000000000000000000 ) ) ;
#4535=CIRCLE ( 'NONE', #294, 7.500000000000000000 ) ;
#4537=AXIS2_PLACEMENT_3D ( 'NONE', #1462, #1696, #8851 ) ;
#4539=ORIENTED_EDGE ( 'NONE', *, *, #13068, .F. ) ;
#4548=ADVANCED_FACE ( 'NONE', ( #12357 ), #1067, .T. ) ;
#4558=CIRCLE ( 'NONE', #3385, 7.500000000000002665 ) ;
#4563=CARTESIAN_POINT ( 'NONE',  ( 7.499999999999999112, 0.000000000000000000, -100.0000000000000000 ) ) ;
#4567=CARTESIAN_POINT ( 'NONE',  ( -130.4031948627971076, -44.80746418436799416, -90.00000000000000000 ) ) ;
#4569=EDGE_CURVE ( 'NONE', #21305, #13461, #20628, .T. ) ;
#4571=AXIS2_PLACEMENT_3D ( 'NONE', #1784, #229, #9662 ) ;
#4613=VECTOR ( 'NONE', #4514, 1000.000000000000000 ) ;
#4631=ORIENTED_EDGE ( 'NONE', *, *, #1244, .T. ) ;
#4637=CARTESIAN_POINT ( 'NONE',  ( -121.5574576620393970, -79.04925354955290118, -2.775557561562891351E-14 ) ) ;
#4660=DIRECTION ( 'NONE',  ( 1.000000000000000000, 0.000000000000000000, 0.000000000000000000 ) ) ;
#4685=CARTESIAN_POINT ( 'NONE',  ( -140.0355749532211007, 37.61698748598567477, 90.00000000000000000 ) ) ;
#4735=ORIENTED_EDGE ( 'NONE', *, *, #1244, .F. ) ;
#4752=CARTESIAN_POINT ( 'NONE',  ( -137.9031948627971076, -44.80746418436799416, 90.00000000000000000 ) ) ;
#4754=VERTEX_POINT ( 'NONE', #9611 ) ;
#4759=EDGE_CURVE ( 'NONE', #5473, #13664, #21188, .T. ) ;
#4763=DIRECTION ( 'NONE',  ( 1.000000000000000000, 0.000000000000000000, 0.000000000000000000 ) ) ;
#4782=EDGE_CURVE ( 'NONE', #6740, #13908, #2884, .T. ) ;
#4786=CARTESIAN_POINT ( 'NONE',  ( -7.499999999999999112, 0.000000000000000000, -100.0000000000000000 ) ) ;
#4790=ADVANCED_FACE ( 'NONE', ( #17337 ), #4521, .F. ) ;
#4806=DIRECTION ( 'NONE',  ( -0.000000000000000000, 0.000000000000000000, -1.000000000000000000 ) ) ;
#4807=ORIENTED_EDGE ( 'NONE', *, *, #18145, .F. ) ;
#4842=ORIENTED_EDGE ( 'NONE', *, *, #21593, .F. ) ;
#4875=DIRECTION ( 'NONE',  ( 0.000000000000000000, 0.000000000000000000, 1.000000000000000000 ) ) ;
#4884=DIRECTION ( 'NONE',  ( 0.000000000000000000, -0.000000000000000000, 1.000000000000000000 ) ) ;
#4918=DIRECTION ( 'NONE',  ( 0.000000000000000000, 0.000000000000000000, 1.000000000000000000 ) ) ;
#4923=DIRECTION ( 'NONE',  ( -0.000000000000000000, 1.000000000000000000, 0.000000000000000000 ) ) ;
#4924=ORIENTED_EDGE ( 'NONE', *, *, #8154, .F. ) ;
#4927=DIRECTION ( 'NONE',  ( -3.700743415417187942E-15, 1.000000000000000000, 0.000000000000000000 ) ) ;
#4933=AXIS2_PLACEMENT_3D ( 'NONE', #14102, #10595, #3650 ) ;
#4937=VERTEX_POINT ( 'NONE', #12288 ) ;
#4943=DIRECTION ( 'NONE',  ( -0.8090169943749507819, 0.5877852522924686962, 0.000000000000000000 ) ) ;
#4959=AXIS2_PLACEMENT_3D ( 'NONE', #15194, #2121, #22885 ) ;
#4971=CIRCLE ( 'NONE', #17321, 7.500000000000002665 ) ;
#4977=DIRECTION ( 'NONE',  ( 0.000000000000000000, 0.000000000000000000, 1.000000000000000000 ) ) ;
#4987=FACE_OUTER_BOUND ( 'NONE', #19860, .T. ) ;
#4997=ORIENTED_EDGE ( 'NONE', *, *, #13396, .T. ) ;
#4998=EDGE_CURVE ( 'NONE', #5086, #10931, #9102, .T. ) ;
#5000=DIRECTION ( 'NONE',  ( 0.000000000000000000, 0.000000000000000000, 1.000000000000000000 ) ) ;
#5023=DIRECTION ( 'NONE',  ( -0.9510565162951557516, 0.3090169943749406234, 0.000000000000000000 ) ) ;
#5027=DIRECTION ( 'NONE',  ( -0.000000000000000000, -0.000000000000000000, 1.000000000000000000 ) ) ;
#5034=CIRCLE ( 'NONE', #16228, 7.500000000000002665 ) ;
#5050=EDGE_CURVE ( 'NONE', #17172, #5473, #20265, .T. ) ;
#5086=VERTEX_POINT ( 'NONE', #20086 ) ;
#5097=DIRECTION ( 'NONE',  ( 0.000000000000000000, 0.000000000000000000, 1.000000000000000000 ) ) ;
#5103=AXIS2_PLACEMENT_3D ( 'NONE', #3974, #11388, #2164 ) ;
#5125=DIRECTION ( 'NONE',  ( -0.000000000000000000, -0.000000000000000000, 1.000000000000000000 ) ) ;
#5128=CARTESIAN_POINT ( 'NONE',  ( 137.9031948627977044, -44.80746418436605438, 90.00000000000000000 ) ) ;
#5147=LINE ( 'NONE', #19985, #7654 ) ;
#5148=AXIS2_PLACEMENT_3D ( 'NONE', #7883, #6305, #19333 ) ;
#5159=EDGE_LOOP ( 'NONE', ( #22553, #4290, #12848, #10050 ) ) ;
#5168=DIRECTION ( 'NONE',  ( 0.000000000000000000, 0.000000000000000000, 1.000000000000000000 ) ) ;
#5181=ORIENTED_EDGE ( 'NONE', *, *, #22626, .F. ) ;
#5182=EDGE_LOOP ( 'NONE', ( #12131, #9938, #6429, #12883 ) ) ;
#5194=ADVANCED_FACE ( 'NONE', ( #7157 ), #11532, .F. ) ;
#5214=ADVANCED_FACE ( 'NONE', ( #17423 ), #2187, .F. ) ;
#5228=CIRCLE ( 'NONE', #18315, 160.0000000000000000 ) ;
#5242=CARTESIAN_POINT ( 'NONE',  ( -7.499999999999999112, 34.18698582794336716, 100.0000000000000000 ) ) ;
#5244=DIRECTION ( 'NONE',  ( 0.000000000000000000, 0.000000000000000000, -1.000000000000000000 ) ) ;
#5259=FACE_OUTER_BOUND ( 'NONE', #23081, .T. ) ;
#5263=CARTESIAN_POINT ( 'NONE',  ( 0.000000000000000000, 0.000000000000000000, -90.00000000000000000 ) ) ;
#5276=ORIENTED_EDGE ( 'NONE', *, *, #9577, .F. ) ;
#5289=DIRECTION ( 'NONE',  ( -0.5877852522924643663, -0.8090169943749537795, 0.000000000000000000 ) ) ;
#5293=ORIENTED_EDGE ( 'NONE', *, *, #22472, .T. ) ;
#5296=VECTOR ( 'NONE', #22077, 1000.000000000000000 ) ;
#5336=ORIENTED_EDGE ( 'NONE', *, *, #9820, .F. ) ;
#5347=CIRCLE ( 'NONE', #23073, 7.500000000000002665 ) ;
#5349=CARTESIAN_POINT ( 'NONE',  ( -79.04925354955248906, 121.5574576620396812, -90.00000000000000000 ) ) ;
#5357=CARTESIAN_POINT ( 'NONE',  ( -160.0000000000000000, 0.000000000000000000, 100.0000000000000000 ) ) ;
#5368=CIRCLE ( 'NONE', #18842, 145.0000000000000284 ) ;
#5399=DIRECTION ( 'NONE',  ( 1.000000000000000000, 0.000000000000000000, 0.000000000000000000 ) ) ;
#5430=AXIS2_PLACEMENT_3D ( 'NONE', #23089, #8257, #19455 ) ;
#5462=ADVANCED_FACE ( 'NONE', ( #8597 ), #23431, .T. ) ;
#5473=VERTEX_POINT ( 'NONE', #7242 ) ;
#5481=ORIENTED_EDGE ( 'NONE', *, *, #2601, .F. ) ;
#5489=CIRCLE ( 'NONE', #2001, 7.500000000000002665 ) ;
#5499=CARTESIAN_POINT ( 'NONE',  ( 51.87806360044628917, 135.4018704341563080, -2.775557561562891351E-14 ) ) ;
#5515=DIRECTION ( 'NONE',  ( -0.000000000000000000, -0.000000000000000000, 1.000000000000000000 ) ) ;
#5520=AXIS2_PLACEMENT_3D ( 'NONE', #15763, #8386, #11695 ) ;
#5554=AXIS2_PLACEMENT_3D ( 'NONE', #2826, #796, #4527 ) ;
#5564=CARTESIAN_POINT ( 'NONE',  ( 0.000000000000000000, 0.000000000000000000, -90.00000000000000000 ) ) ;
#5569=ORIENTED_EDGE ( 'NONE', *, *, #6770, .F. ) ;
#5575=EDGE_LOOP ( 'NONE', ( #23599, #7158, #7140, #20153 ) ) ;
#5586=ORIENTED_EDGE ( 'NONE', *, *, #21071, .F. ) ;
#5588=CIRCLE ( 'NONE', #19073, 7.500000000000002665 ) ;
#5609=AXIS2_PLACEMENT_3D ( 'NONE', #6745, #8320, #13920 ) ;
#5648=DIRECTION ( 'NONE',  ( -0.000000000000000000, -0.000000000000000000, 1.000000000000000000 ) ) ;
#5651=VERTEX_POINT ( 'NONE', #13692 ) ;
#5656=FACE_OUTER_BOUND ( 'NONE', #17417, .T. ) ;
#5701=DIRECTION ( 'NONE',  ( -3.700743415417187942E-15, 1.000000000000000000, 0.000000000000000000 ) ) ;
#5721=DIRECTION ( 'NONE',  ( -1.000000000000000000, 0.000000000000000000, 0.000000000000000000 ) ) ;
#5742=CIRCLE ( 'NONE', #9221, 35.00000000000000711 ) ;
#5758=DIRECTION ( 'NONE',  ( -0.000000000000000000, -0.000000000000000000, 1.000000000000000000 ) ) ;
#5759=ORIENTED_EDGE ( 'NONE', *, *, #14624, .T. ) ;
#5762=CYLINDRICAL_SURFACE ( 'NONE', #8124, 35.00000000000000711 ) ;
#5790=FACE_BOUND ( 'NONE', #22978, .T. ) ;
#5797=FACE_OUTER_BOUND ( 'NONE', #19410, .T. ) ;
#5811=ORIENTED_EDGE ( 'NONE', *, *, #23434, .F. ) ;
#5818=VERTEX_POINT ( 'NONE', #1316 ) ;
#5827=ORIENTED_EDGE ( 'NONE', *, *, #3694, .F. ) ;
#5828=DIRECTION ( 'NONE',  ( 0.000000000000000000, 0.000000000000000000, 1.000000000000000000 ) ) ;
#5831=FACE_OUTER_BOUND ( 'NONE', #15927, .T. ) ;
#5841=ORIENTED_EDGE ( 'NONE', *, *, #8556, .T. ) ;
#5874=DIRECTION ( 'NONE',  ( 0.000000000000000000, 0.000000000000000000, 1.000000000000000000 ) ) ;
#5910=ORIENTED_EDGE ( 'NONE', *, *, #11723, .T. ) ;
#5917=EDGE_CURVE ( 'NONE', #10526, #11121, #16600, .T. ) ;
#5924=EDGE_CURVE ( 'NONE', #10981, #3142, #1565, .T. ) ;
#5942=ORIENTED_EDGE ( 'NONE', *, *, #20073, .T. ) ;
#5963=CARTESIAN_POINT ( 'NONE',  ( -112.7436279071531828, 91.18044947428914782, -2.775557561562891351E-14 ) ) ;
#5964=ORIENTED_EDGE ( 'NONE', *, *, #12059, .T. ) ;
#5965=DIRECTION ( 'NONE',  ( 1.000000000000000000, 0.000000000000000000, 0.000000000000000000 ) ) ;
#5992=ORIENTED_EDGE ( 'NONE', *, *, #4998, .F. ) ;
#6014=ORIENTED_EDGE ( 'NONE', *, *, #8841, .F. ) ;
#6017=AXIS2_PLACEMENT_3D ( 'NONE', #22251, #14922, #3906 ) ;
#6035=DIRECTION ( 'NONE',  ( 0.000000000000000000, -0.000000000000000000, 1.000000000000000000 ) ) ;
#6043=AXIS2_PLACEMENT_3D ( 'NONE', #6819, #16126, #9442 ) ;
#6046=CIRCLE ( 'NONE', #10720, 145.0000000000000284 ) ;
#6076=CYLINDRICAL_SURFACE ( 'NONE', #22755, 145.0000000000000284 ) ;
#6080=CYLINDRICAL_SURFACE ( 'NONE', #6017, 7.500000000000007105 ) ;
#6100=AXIS2_PLACEMENT_3D ( 'NONE', #20679, #11313, #18622 ) ;
#6104=CARTESIAN_POINT ( 'NONE',  ( -117.3074641843675749, 85.22886158240835641, 90.00000000000000000 ) ) ;
#6105=AXIS2_PLACEMENT_3D ( 'NONE', #22951, #19095, #6423 ) ;
#6145=AXIS2_PLACEMENT_3D ( 'NONE', #669, #14306, #21642 ) ;
#6155=ORIENTED_EDGE ( 'NONE', *, *, #2777, .T. ) ;
#6165=VECTOR ( 'NONE', #10576, 1000.000000000000000 ) ;
#6169=EDGE_CURVE ( 'NONE', #4516, #11736, #821, .T. ) ;
#6173=ORIENTED_EDGE ( 'NONE', *, *, #23531, .T. ) ;
#6182=AXIS2_PLACEMENT_3D ( 'NONE', #19789, #3239, #10651 ) ;
#6188=CYLINDRICAL_SURFACE ( 'NONE', #16495, 160.0000000000000000 ) ;
#6206=VERTEX_POINT ( 'NONE', #4685 ) ;
#6209=CYLINDRICAL_SURFACE ( 'NONE', #417, 7.500000000000007105 ) ;
#6215=EDGE_CURVE ( 'NONE', #13931, #3378, #5034, .T. ) ;
#6228=LINE ( 'NONE', #4031, #21163 ) ;
#6230=CARTESIAN_POINT ( 'NONE',  ( 0.000000000000000000, 0.000000000000000000, -90.00000000000000000 ) ) ;
#6233=CARTESIAN_POINT ( 'NONE',  ( -137.9031948627971076, -44.80746418436799416, 90.00000000000000000 ) ) ;
#6239=EDGE_CURVE ( 'NONE', #13321, #10209, #20395, .T. ) ;
#6244=CARTESIAN_POINT ( 'NONE',  ( -35.00000000000000711, 4.286263797015737285E-15, -100.0000000000000000 ) ) ;
#6251=CARTESIAN_POINT ( 'NONE',  ( 0.000000000000000000, 0.000000000000000000, 90.00000000000000000 ) ) ;
#6287=ORIENTED_EDGE ( 'NONE', *, *, #6495, .F. ) ;
#6305=DIRECTION ( 'NONE',  ( 0.000000000000000000, 0.000000000000000000, 1.000000000000000000 ) ) ;
#6313=AXIS2_PLACEMENT_3D ( 'NONE', #6104, #12073, #13526 ) ;
#6342=CYLINDRICAL_SURFACE ( 'NONE', #20760, 145.0000000000000284 ) ;
#6351=DIRECTION ( 'NONE',  ( 0.000000000000000000, 0.000000000000000000, 1.000000000000000000 ) ) ;
#6358=CYLINDRICAL_SURFACE ( 'NONE', #16306, 145.0000000000000284 ) ;
#6361=EDGE_CURVE ( 'NONE', #18342, #880, #19248, .T. ) ;
#6362=ORIENTED_EDGE ( 'NONE', *, *, #2318, .T. ) ;
#6364=CARTESIAN_POINT ( 'NONE',  ( 79.04925354955072692, 121.5574576620408322, -90.00000000000000000 ) ) ;
#6377=VECTOR ( 'NONE', #16983, 1000.000000000000000 ) ;
#6378=ORIENTED_EDGE ( 'NONE', *, *, #8160, .F. ) ;
#6386=FACE_OUTER_BOUND ( 'NONE', #8801, .T. ) ;
#6404=DIRECTION ( 'NONE',  ( 1.000000000000000000, 0.000000000000000000, 0.000000000000000000 ) ) ;
#6415=DIRECTION ( 'NONE',  ( 0.000000000000000000, 0.000000000000000000, 1.000000000000000000 ) ) ;
#6420=EDGE_LOOP ( 'NONE', ( #20134, #11761, #17500, #10580 ) ) ;
#6423=DIRECTION ( 'NONE',  ( -0.3090169943749517811, 0.9510565162951520879, 0.000000000000000000 ) ) ;
#6424=CARTESIAN_POINT ( 'NONE',  ( -7.499999999999999112, 41.99999999999998579, -100.0000000000000000 ) ) ;
#6429=ORIENTED_EDGE ( 'NONE', *, *, #10475, .F. ) ;
#6433=DIRECTION ( 'NONE',  ( -0.000000000000000000, 0.000000000000000000, -1.000000000000000000 ) ) ;
#6434=CARTESIAN_POINT ( 'NONE',  ( -7.499999999999997335, 34.18698582794336005, -100.0000000000000000 ) ) ;
#6440=DIRECTION ( 'NONE',  ( -0.9510565162951557516, 0.3090169943749406234, 0.000000000000000000 ) ) ;
#6455=CARTESIAN_POINT ( 'NONE',  ( -79.04925354955163641, -121.5574576620402496, 90.00000000000000000 ) ) ;
#6466=EDGE_CURVE ( 'NONE', #7547, #16501, #22329, .T. ) ;
#6479=CIRCLE ( 'NONE', #17661, 145.0000000000000284 ) ;
#6495=EDGE_CURVE ( 'NONE', #18184, #15856, #16989, .T. ) ;
#6511=CARTESIAN_POINT ( 'NONE',  ( 91.18044947428791147, 112.7436279071541776, -2.775557561562891351E-14 ) ) ;
#6538=CARTESIAN_POINT ( 'NONE',  ( -7.497491405671719455, -144.8060344827586334, 90.00000000000000000 ) ) ;
#6546=ORIENTED_EDGE ( 'NONE', *, *, #7064, .T. ) ;
#6551=DIRECTION ( 'NONE',  ( 1.000000000000000000, 0.000000000000000000, 0.000000000000000000 ) ) ;
#6560=CIRCLE ( 'NONE', #10449, 7.500000000000000888 ) ;
#6565=LINE ( 'NONE', #4637, #17771 ) ;
#6591=DIRECTION ( 'NONE',  ( -0.3090169943749370707, -0.9510565162951569729, 0.000000000000000000 ) ) ;
#6600=DIRECTION ( 'NONE',  ( 0.000000000000000000, -0.000000000000000000, -1.000000000000000000 ) ) ;
#6601=EDGE_CURVE ( 'NONE', #4268, #22523, #4204, .T. ) ;
#6630=EDGE_CURVE ( 'NONE', #4114, #13072, #14064, .T. ) ;
#6633=EDGE_CURVE ( 'NONE', #13320, #9308, #16552, .T. ) ;
#6636=DIRECTION ( 'NONE',  ( -0.000000000000000000, -0.000000000000000000, 1.000000000000000000 ) ) ;
#6640=VERTEX_POINT ( 'NONE', #23567 ) ;
#6648=EDGE_CURVE ( 'NONE', #20079, #21672, #17340, .T. ) ;
#6649=ORIENTED_EDGE ( 'NONE', *, *, #4432, .F. ) ;
#6679=FACE_OUTER_BOUND ( 'NONE', #2612, .T. ) ;
#6708=CYLINDRICAL_SURFACE ( 'NONE', #4933, 7.500000000000000888 ) ;
#6723=FACE_OUTER_BOUND ( 'NONE', #13226, .T. ) ;
#6739=CARTESIAN_POINT ( 'NONE',  ( -145.0000000000000284, -5.062647941322544249E-13, 90.00000000000000000 ) ) ;
#6740=VERTEX_POINT ( 'NONE', #134 ) ;
#6745=CARTESIAN_POINT ( 'NONE',  ( -85.22886158240795851, -117.3074641843678876, -90.00000000000000000 ) ) ;
#6761=CARTESIAN_POINT ( 'NONE',  ( -160.0000000000000000, 0.000000000000000000, 90.00000000000000000 ) ) ;
#6770=EDGE_CURVE ( 'NONE', #18600, #14720, #5489, .T. ) ;
#6771=AXIS2_PLACEMENT_3D ( 'NONE', #10398, #17613, #4943 ) ;
#6782=CARTESIAN_POINT ( 'NONE',  ( 0.000000000000000000, 0.000000000000000000, -90.00000000000000000 ) ) ;
#6786=DIRECTION ( 'NONE',  ( 1.000000000000000000, 0.000000000000000000, 0.000000000000000000 ) ) ;
#6798=FACE_OUTER_BOUND ( 'NONE', #501, .T. ) ;
#6808=DIRECTION ( 'NONE',  ( 1.000000000000000000, 0.000000000000000000, 0.000000000000000000 ) ) ;
#6809=ORIENTED_EDGE ( 'NONE', *, *, #1951, .T. ) ;
#6815=FACE_OUTER_BOUND ( 'NONE', #11889, .T. ) ;
#6817=LINE ( 'NONE', #14210, #13516 ) ;
#6819=CARTESIAN_POINT ( 'NONE',  ( 0.000000000000000000, 0.000000000000000000, -90.00000000000000000 ) ) ;
#6839=DIRECTION ( 'NONE',  ( 0.000000000000000000, 0.000000000000000000, -1.000000000000000000 ) ) ;
#6840=ORIENTED_EDGE ( 'NONE', *, *, #23744, .T. ) ;
#6841=AXIS2_PLACEMENT_3D ( 'NONE', #6852, #14253, #17727 ) ;
#6849=FACE_OUTER_BOUND ( 'NONE', #17894, .T. ) ;
#6850=EDGE_LOOP ( 'NONE', ( #8235, #17972, #10146, #15476 ) ) ;
#6852=CARTESIAN_POINT ( 'NONE',  ( 0.000000000000000000, 0.000000000000000000, -90.00000000000000000 ) ) ;
#6853=DIRECTION ( 'NONE',  ( 0.000000000000000000, 0.000000000000000000, 1.000000000000000000 ) ) ;
#6868=EDGE_CURVE ( 'NONE', #13320, #766, #7409, .T. ) ;
#6892=AXIS2_PLACEMENT_3D ( 'NONE', #6233, #2475, #18763 ) ;
#6893=VECTOR ( 'NONE', #22524, 1000.000000000000000 ) ;
#6906=CARTESIAN_POINT ( 'NONE',  ( -140.0355749532208449, -37.61698748598668374, 90.00000000000000000 ) ) ;
#6948=DIRECTION ( 'NONE',  ( 0.000000000000000000, 0.000000000000000000, 1.000000000000000000 ) ) ;
#6965=DIRECTION ( 'NONE',  ( 0.000000000000000000, 0.000000000000000000, -1.000000000000000000 ) ) ;
#6989=LINE ( 'NONE', #16165, #13114 ) ;
#6999=CARTESIAN_POINT ( 'NONE',  ( 37.61698748598717401, -140.0355749532207312, -90.00000000000000000 ) ) ;
#7014=EDGE_CURVE ( 'NONE', #23533, #3375, #20721, .T. ) ;
#7047=ORIENTED_EDGE ( 'NONE', *, *, #22555, .F. ) ;
#7060=AXIS2_PLACEMENT_3D ( 'NONE', #19516, #21236, #19644 ) ;
#7064=EDGE_CURVE ( 'NONE', #18600, #6206, #19146, .T. ) ;
#7066=CARTESIAN_POINT ( 'NONE',  ( 121.5574576620405622, -79.04925354955115324, -2.775557561562891351E-14 ) ) ;
#7074=ADVANCED_FACE ( 'NONE', ( #4185 ), #6358, .T. ) ;
#7082=CARTESIAN_POINT ( 'NONE',  ( -130.4031948627971076, -44.80746418436799416, -90.00000000000000000 ) ) ;
#7084=ORIENTED_EDGE ( 'NONE', *, *, #6239, .F. ) ;
#7090=AXIS2_PLACEMENT_3D ( 'NONE', #3483, #10892, #10760 ) ;
#7107=CARTESIAN_POINT ( 'NONE',  ( -7.499999999999999112, 41.99999999999998579, -100.0000000000000000 ) ) ;
#7136=DIRECTION ( 'NONE',  ( 0.000000000000000000, 0.000000000000000000, 1.000000000000000000 ) ) ;
#7138=DIRECTION ( 'NONE',  ( 0.5877852522924719159, 0.8090169943749482284, 0.000000000000000000 ) ) ;
#7140=ORIENTED_EDGE ( 'NONE', *, *, #18407, .F. ) ;
#7145=ORIENTED_EDGE ( 'NONE', *, *, #7014, .F. ) ;
#7157=FACE_OUTER_BOUND ( 'NONE', #22757, .T. ) ;
#7158=ORIENTED_EDGE ( 'NONE', *, *, #23434, .T. ) ;
#7160=DIRECTION ( 'NONE',  ( 0.000000000000000000, 0.000000000000000000, 1.000000000000000000 ) ) ;
#7169=VERTEX_POINT ( 'NONE', #6761 ) ;
#7176=ORIENTED_EDGE ( 'NONE', *, *, #5917, .F. ) ;
#7192=CIRCLE ( 'NONE', #6043, 145.0000000000000284 ) ;
#7217=EDGE_LOOP ( 'NONE', ( #22701, #22158, #22464, #13916 ) ) ;
#7226=AXIS2_PLACEMENT_3D ( 'NONE', #452, #15189, #9993 ) ;
#7232=DIRECTION ( 'NONE',  ( 0.000000000000000000, 0.000000000000000000, 1.000000000000000000 ) ) ;
#7242=CARTESIAN_POINT ( 'NONE',  ( 7.499999999999997335, 34.18698582794336005, 100.0000000000000000 ) ) ;
#7243=EDGE_CURVE ( 'NONE', #17692, #6740, #16195, .T. ) ;
#7273=EDGE_LOOP ( 'NONE', ( #4842, #16571, #9538, #11746 ) ) ;
#7287=LINE ( 'NONE', #10709, #10788 ) ;
#7291=AXIS2_PLACEMENT_3D ( 'NONE', #9943, #517, #18723 ) ;
#7292=AXIS2_PLACEMENT_3D ( 'NONE', #13452, #13809, #6404 ) ;
#7329=CARTESIAN_POINT ( 'NONE',  ( -130.4031948627974486, 44.80746418436699940, -90.00000000000000000 ) ) ;
#7352=ORIENTED_EDGE ( 'NONE', *, *, #835, .T. ) ;
#7370=ADVANCED_FACE ( 'NONE', ( #22186 ), #21836, .F. ) ;
#7409=CIRCLE ( 'NONE', #5103, 7.499999999999996447 ) ;
#7440=ORIENTED_EDGE ( 'NONE', *, *, #12332, .F. ) ;
#7476=AXIS2_PLACEMENT_3D ( 'NONE', #14680, #20444, #22019 ) ;
#7490=ORIENTED_EDGE ( 'NONE', *, *, #23744, .F. ) ;
#7495=EDGE_LOOP ( 'NONE', ( #18483, #20018, #680, #13342 ) ) ;
#7505=ORIENTED_EDGE ( 'NONE', *, *, #20105, .F. ) ;
#7531=CARTESIAN_POINT ( 'NONE',  ( 0.000000000000000000, 0.000000000000000000, -90.00000000000000000 ) ) ;
#7535=AXIS2_PLACEMENT_3D ( 'NONE', #16665, #7232, #119 ) ;
#7547=VERTEX_POINT ( 'NONE', #4197 ) ;
#7548=CARTESIAN_POINT ( 'NONE',  ( 7.497491405671719455, 144.8060344827586334, -2.775557561562891351E-14 ) ) ;
#7550=AXIS2_PLACEMENT_3D ( 'NONE', #12962, #3723, #20387 ) ;
#7574=DIRECTION ( 'NONE',  ( 1.000000000000000000, 0.000000000000000000, 0.000000000000000000 ) ) ;
#7615=VERTEX_POINT ( 'NONE', #10379 ) ;
#7625=ORIENTED_EDGE ( 'NONE', *, *, #14939, .T. ) ;
#7632=AXIS2_PLACEMENT_3D ( 'NONE', #14719, #4177, #329 ) ;
#7634=VERTEX_POINT ( 'NONE', #10140 ) ;
#7640=CARTESIAN_POINT ( 'NONE',  ( 0.000000000000000000, 0.000000000000000000, 90.00000000000000000 ) ) ;
#7644=CIRCLE ( 'NONE', #9593, 7.499999999999996447 ) ;
#7647=VECTOR ( 'NONE', #5244, 1000.000000000000000 ) ;
#7650=EDGE_CURVE ( 'NONE', #13664, #10493, #16040, .T. ) ;
#7654=VECTOR ( 'NONE', #19873, 1000.000000000000000 ) ;
#7657=ADVANCED_FACE ( 'NONE', ( #6849 ), #8310, .F. ) ;
#7661=ORIENTED_EDGE ( 'NONE', *, *, #21593, .T. ) ;
#7671=DIRECTION ( 'NONE',  ( -0.000000000000000000, -0.000000000000000000, 1.000000000000000000 ) ) ;
#7675=CARTESIAN_POINT ( 'NONE',  ( 37.61698748598424658, 140.0355749532214986, -2.775557561562891351E-14 ) ) ;
#7691=AXIS2_PLACEMENT_3D ( 'NONE', #23677, #18018, #7138 ) ;
#7717=COLOUR_RGB ( '',0.8941176470588234615, 0.8941176470588234615, 0.8941176470588234615 ) ;
#7721=AXIS2_PLACEMENT_3D ( 'NONE', #17394, #22025, #11549 ) ;
#7778=DIRECTION ( 'NONE',  ( -0.000000000000000000, -0.000000000000000000, -1.000000000000000000 ) ) ;
#7780=DIRECTION ( 'NONE',  ( 1.000000000000000000, 0.000000000000000000, 0.000000000000000000 ) ) ;
#7813=CYLINDRICAL_SURFACE ( 'NONE', #8051, 7.500000000000000000 ) ;
#7817=DIRECTION ( 'NONE',  ( -0.000000000000000000, -0.000000000000000000, 1.000000000000000000 ) ) ;
#7820=CARTESIAN_POINT ( 'NONE',  ( -91.18044947428874991, -112.7436279071535097, -2.775557561562891351E-14 ) ) ;
#7827=SHAPE_DEFINITION_REPRESENTATION ( #1492, #8847 ) ;
#7863=ORIENTED_EDGE ( 'NONE', *, *, #13767, .F. ) ;
#7864=DIRECTION ( 'NONE',  ( -0.000000000000000000, 0.000000000000000000, 1.000000000000000000 ) ) ;
#7883=CARTESIAN_POINT ( 'NONE',  ( -145.0000000000000284, -5.062647941322544249E-13, 90.00000000000000000 ) ) ;
#7888=DIRECTION ( 'NONE',  ( -0.000000000000000000, -0.000000000000000000, 1.000000000000000000 ) ) ;
#7919=CIRCLE ( 'NONE', #11029, 7.500000000000003553 ) ;
#7920=DIRECTION ( 'NONE',  ( 1.000000000000000000, 0.000000000000000000, 0.000000000000000000 ) ) ;
#7940=CARTESIAN_POINT ( 'NONE',  ( -121.5574576620399654, 79.04925354955206274, 90.00000000000000000 ) ) ;
#7958=DIRECTION ( 'NONE',  ( 1.000000000000000000, 0.000000000000000000, 0.000000000000000000 ) ) ;
#7975=LINE ( 'NONE', #383, #16731 ) ;
#7988=CIRCLE ( 'NONE', #1794, 7.500000000000005329 ) ;
#8030=ORIENTED_EDGE ( 'NONE', *, *, #22440, .T. ) ;
#8034=EDGE_CURVE ( 'NONE', #11303, #2320, #19390, .T. ) ;
#8035=CARTESIAN_POINT ( 'NONE',  ( 137.9031948627977044, -44.80746418436605438, -90.00000000000000000 ) ) ;
#8036=ORIENTED_EDGE ( 'NONE', *, *, #3305, .F. ) ;
#8042=CARTESIAN_POINT ( 'NONE',  ( 135.4018704341561374, -51.87806360044677234, 90.00000000000000000 ) ) ;
#8044=CIRCLE ( 'NONE', #9198, 145.0000000000000284 ) ;
#8051=AXIS2_PLACEMENT_3D ( 'NONE', #9998, #807, #18913 ) ;
#8072=CARTESIAN_POINT ( 'NONE',  ( 0.000000000000000000, 0.000000000000000000, -100.0000000000000000 ) ) ;
#8107=ORIENTED_EDGE ( 'NONE', *, *, #6466, .T. ) ;
#8120=CIRCLE ( 'NONE', #15012, 7.500000000000004441 ) ;
#8124=AXIS2_PLACEMENT_3D ( 'NONE', #3471, #5515, #16394 ) ;
#8126=VERTEX_POINT ( 'NONE', #3182 ) ;
#8130=CARTESIAN_POINT ( 'NONE',  ( -117.3074641843669781, -85.22886158240918064, -90.00000000000000000 ) ) ;
#8134=FACE_OUTER_BOUND ( 'NONE', #3958, .T. ) ;
#8138=ORIENTED_EDGE ( 'NONE', *, *, #15235, .F. ) ;
#8140=FACE_OUTER_BOUND ( 'NONE', #5575, .T. ) ;
#8154=EDGE_CURVE ( 'NONE', #9872, #11044, #7192, .T. ) ;
#8160=EDGE_CURVE ( 'NONE', #12572, #4754, #16457, .T. ) ;
#8164=DIRECTION ( 'NONE',  ( -0.000000000000000000, 0.000000000000000000, -1.000000000000000000 ) ) ;
#8173=DIRECTION ( 'NONE',  ( 1.000000000000000000, 0.000000000000000000, 0.000000000000000000 ) ) ;
#8178=EDGE_LOOP ( 'NONE', ( #15258, #23028, #17791, #15730 ) ) ;
#8184=FACE_OUTER_BOUND ( 'NONE', #2760, .T. ) ;
#8185=DIRECTION ( 'NONE',  ( 1.000000000000000000, 0.000000000000000000, 0.000000000000000000 ) ) ;
#8196=DIRECTION ( 'NONE',  ( 0.000000000000000000, 0.000000000000000000, 1.000000000000000000 ) ) ;
#8200=DIRECTION ( 'NONE',  ( 1.000000000000000000, 0.000000000000000000, 0.000000000000000000 ) ) ;
#8227=VECTOR ( 'NONE', #4923, 1000.000000000000000 ) ;
#8235=ORIENTED_EDGE ( 'NONE', *, *, #8556, .F. ) ;
#8252=ORIENTED_EDGE ( 'NONE', *, *, #3031, .F. ) ;
#8257=DIRECTION ( 'NONE',  ( 0.000000000000000000, 0.000000000000000000, 1.000000000000000000 ) ) ;
#8292=LINE ( 'NONE', #8403, #21936 ) ;
#8304=DIRECTION ( 'NONE',  ( 1.000000000000000000, 0.000000000000000000, 0.000000000000000000 ) ) ;
#8310=CYLINDRICAL_SURFACE ( 'NONE', #7060, 7.500000000000007105 ) ;
#8317=ORIENTED_EDGE ( 'NONE', *, *, #13798, .T. ) ;
#8318=CIRCLE ( 'NONE', #13349, 7.500000000000004441 ) ;
#8320=DIRECTION ( 'NONE',  ( 0.000000000000000000, -0.000000000000000000, 1.000000000000000000 ) ) ;
#8330=DIRECTION ( 'NONE',  ( 1.000000000000000000, 0.000000000000000000, 0.000000000000000000 ) ) ;
#8347=CARTESIAN_POINT ( 'NONE',  ( -144.8060344827586619, 7.497491405671214082, -90.00000000000000000 ) ) ;
#8356=DIRECTION ( 'NONE',  ( -0.000000000000000000, -0.000000000000000000, 1.000000000000000000 ) ) ;
#8358=ADVANCED_FACE ( 'NONE', ( #8823 ), #14399, .F. ) ;
#8375=CIRCLE ( 'NONE', #19931, 145.0000000000000284 ) ;
#8386=DIRECTION ( 'NONE',  ( 0.000000000000000000, 0.000000000000000000, 1.000000000000000000 ) ) ;
#8397=DIRECTION ( 'NONE',  ( -0.000000000000000000, -0.000000000000000000, 1.000000000000000000 ) ) ;
#8398=DIRECTION ( 'NONE',  ( 1.000000000000000000, 0.000000000000000000, 0.000000000000000000 ) ) ;
#8403=CARTESIAN_POINT ( 'NONE',  ( 79.04925354955338435, -121.5574576620390843, -2.775557561562891351E-14 ) ) ;
#8405=EDGE_CURVE ( 'NONE', #7615, #13673, #8375, .T. ) ;
#8418=VECTOR ( 'NONE', #21685, 1000.000000000000000 ) ;
#8421=ORIENTED_EDGE ( 'NONE', *, *, #3545, .T. ) ;
#8424=DIRECTION ( 'NONE',  ( -0.000000000000000000, -0.000000000000000000, 1.000000000000000000 ) ) ;
#8440=AXIS2_PLACEMENT_3D ( 'NONE', #12886, #18612, #14438 ) ;
#8443=CIRCLE ( 'NONE', #18074, 145.0000000000000284 ) ;
#8455=ORIENTED_EDGE ( 'NONE', *, *, #3241, .T. ) ;
#8469=ORIENTED_EDGE ( 'NONE', *, *, #15968, .T. ) ;
#8479=VECTOR ( 'NONE', #14927, 1000.000000000000000 ) ;
#8484=FACE_OUTER_BOUND ( 'NONE', #10415, .T. ) ;
#8503=CYLINDRICAL_SURFACE ( 'NONE', #8844, 7.500000000000000000 ) ;
#8507=CARTESIAN_POINT ( 'NONE',  ( -91.18044947428953151, 112.7436279071528702, -90.00000000000000000 ) ) ;
#8508=ORIENTED_EDGE ( 'NONE', *, *, #8160, .T. ) ;
#8511=DIRECTION ( 'NONE',  ( 0.000000000000000000, 0.000000000000000000, 1.000000000000000000 ) ) ;
#8524=CARTESIAN_POINT ( 'NONE',  ( 0.000000000000000000, 0.000000000000000000, 100.0000000000000000 ) ) ;
#8556=EDGE_CURVE ( 'NONE', #22764, #11081, #9176, .T. ) ;
#8585=ADVANCED_FACE ( 'NONE', ( #17027 ), #19045, .T. ) ;
#8591=ORIENTED_EDGE ( 'NONE', *, *, #18170, .F. ) ;
#8595=LINE ( 'NONE', #10297, #16768 ) ;
#8597=FACE_OUTER_BOUND ( 'NONE', #9188, .T. ) ;
#8627=ORIENTED_EDGE ( 'NONE', *, *, #9935, .T. ) ;
#8630=ORIENTED_EDGE ( 'NONE', *, *, #23531, .F. ) ;
#8633=CIRCLE ( 'NONE', #7090, 7.499999999999998224 ) ;
#8639=ORIENTED_EDGE ( 'NONE', *, *, #11142, .F. ) ;
#8675=VERTEX_POINT ( 'NONE', #9778 ) ;
#8693=ORIENTED_EDGE ( 'NONE', *, *, #4109, .T. ) ;
#8703=AXIS2_PLACEMENT_3D ( 'NONE', #17389, #18934, #7958 ) ;
#8732=EDGE_LOOP ( 'NONE', ( #5276, #13813, #23184, #21223 ) ) ;
#8735=LINE ( 'NONE', #9212, #15055 ) ;
#8739=CARTESIAN_POINT ( 'NONE',  ( 144.8060344827587187, -7.497491405670202447, -90.00000000000000000 ) ) ;
#8740=EDGE_CURVE ( 'NONE', #1295, #21317, #16045, .T. ) ;
#8745=ADVANCED_FACE ( 'NONE', ( #10260 ), #1053, .T. ) ;
#8773=AXIS2_PLACEMENT_3D ( 'NONE', #17393, #4338, #13921 ) ;
#8775=DIRECTION ( 'NONE',  ( 1.000000000000000000, 0.000000000000000000, 0.000000000000000000 ) ) ;
#8783=EDGE_CURVE ( 'NONE', #3110, #9858, #23788, .T. ) ;
#8785=ORIENTED_EDGE ( 'NONE', *, *, #17170, .T. ) ;
#8791=DIRECTION ( 'NONE',  ( 1.000000000000000000, 0.000000000000000000, 0.000000000000000000 ) ) ;
#8798=EDGE_LOOP ( 'NONE', ( #20347, #4489, #13008, #10684 ) ) ;
#8801=EDGE_LOOP ( 'NONE', ( #2185, #20140, #16234, #14079 ) ) ;
#8806=DIRECTION ( 'NONE',  ( 0.000000000000000000, 0.000000000000000000, 1.000000000000000000 ) ) ;
#8823=FACE_OUTER_BOUND ( 'NONE', #21564, .T. ) ;
#8838=CIRCLE ( 'NONE', #19229, 7.500000000000003553 ) ;
#8841=EDGE_CURVE ( 'NONE', #21770, #22523, #14960, .T. ) ;
#8844=AXIS2_PLACEMENT_3D ( 'NONE', #17907, #21295, #15877 ) ;
#8847=SHAPE_REPRESENTATION ( 'head pulley', ( #11210 ), #17342 ) ;
#8851=DIRECTION ( 'NONE',  ( -1.000000000000000000, 0.000000000000000000, 0.000000000000000000 ) ) ;
#8871=ORIENTED_EDGE ( 'NONE', *, *, #6495, .T. ) ;
#8874=CARTESIAN_POINT ( 'NONE',  ( -37.30746418436648071, -137.9031948627975908, 90.00000000000000000 ) ) ;
#8923=APPLICATION_CONTEXT ( 'automotive_design' ) ;
#8935=EDGE_CURVE ( 'NONE', #21483, #11736, #19947, .T. ) ;
#8961=DIRECTION ( 'NONE',  ( 1.000000000000000000, 0.000000000000000000, 0.000000000000000000 ) ) ;
#8962=ORIENTED_EDGE ( 'NONE', *, *, #20230, .T. ) ;
#8980=EDGE_CURVE ( 'NONE', #11081, #1322, #23048, .T. ) ;
#8996=CARTESIAN_POINT ( 'NONE',  ( 91.18044947429038416, -112.7436279071521881, 90.00000000000000000 ) ) ;
#9002=AXIS2_PLACEMENT_3D ( 'NONE', #10342, #2829, #13992 ) ;
#9011=DIRECTION ( 'NONE',  ( -0.000000000000000000, -0.000000000000000000, 1.000000000000000000 ) ) ;
#9030=DIRECTION ( 'NONE',  ( -0.9510565162951510887, -0.3090169943749553894, 0.000000000000000000 ) ) ;
#9032=ORIENTED_EDGE ( 'NONE', *, *, #10465, .F. ) ;
#9076=AXIS2_PLACEMENT_3D ( 'NONE', #11739, #13309, #19046 ) ;
#9085=AXIS2_PLACEMENT_3D ( 'NONE', #11810, #9736, #19123 ) ;
#9102=CIRCLE ( 'NONE', #3291, 160.0000000000000000 ) ;
#9103=ORIENTED_EDGE ( 'NONE', *, *, #2944, .F. ) ;
#9109=ADVANCED_FACE ( 'NONE', ( #15309 ), #9506, .F. ) ;
#9115=SURFACE_STYLE_FILL_AREA ( #16826 ) ;
#9121=ORIENTED_EDGE ( 'NONE', *, *, #20620, .T. ) ;
#9161=DIRECTION ( 'NONE',  ( 0.000000000000000000, 0.000000000000000000, 1.000000000000000000 ) ) ;
#9176=LINE ( 'NONE', #20379, #3350 ) ;
#9186=CARTESIAN_POINT ( 'NONE',  ( 35.00000000000000711, 0.000000000000000000, -100.0000000000000000 ) ) ;
#9188=EDGE_LOOP ( 'NONE', ( #7047, #16267, #8591, #14492 ) ) ;
#9198=AXIS2_PLACEMENT_3D ( 'NONE', #21509, #21988, #3152 ) ;
#9204=CARTESIAN_POINT ( 'NONE',  ( -112.7436279071531828, 91.18044947428913360, 90.00000000000000000 ) ) ;
#9212=CARTESIAN_POINT ( 'NONE',  ( -109.8074641843675749, 85.22886158240835641, -90.00000000000000000 ) ) ;
#9221=AXIS2_PLACEMENT_3D ( 'NONE', #20936, #19237, #11801 ) ;
#9224=AXIS2_PLACEMENT_3D ( 'NONE', #5564, #3976, #2165 ) ;
#9242=CIRCLE ( 'NONE', #10034, 145.0000000000000284 ) ;
#9243=CIRCLE ( 'NONE', #13889, 145.0000000000000284 ) ;
#9255=DIRECTION ( 'NONE',  ( 1.000000000000000000, 0.000000000000000000, 0.000000000000000000 ) ) ;
#9256=LINE ( 'NONE', #2094, #8479 ) ;
#9275=PRODUCT_DEFINITION_FORMATION_WITH_SPECIFIED_SOURCE ( 'ANY', '', #20003, .NOT_KNOWN. ) ;
#9282=VECTOR ( 'NONE', #5758, 1000.000000000000000 ) ;
#9284=CARTESIAN_POINT ( 'NONE',  ( -117.3074641843675749, 85.22886158240835641, -90.00000000000000000 ) ) ;
#9290=ADVANCED_FACE ( 'NONE', ( #23237 ), #6708, .F. ) ;
#9295=DIRECTION ( 'NONE',  ( 0.000000000000000000, 0.000000000000000000, 1.000000000000000000 ) ) ;
#9308=VERTEX_POINT ( 'NONE', #14688 ) ;
#9321=VERTEX_POINT ( 'NONE', #16360 ) ;
#9340=ORIENTED_EDGE ( 'NONE', *, *, #20939, .T. ) ;
#9346=DIRECTION ( 'NONE',  ( 0.000000000000000000, 0.000000000000000000, 1.000000000000000000 ) ) ;
#9352=DIRECTION ( 'NONE',  ( -0.000000000000000000, -0.000000000000000000, 1.000000000000000000 ) ) ;
#9363=ORIENTED_EDGE ( 'NONE', *, *, #15942, .T. ) ;
#9371=VERTEX_POINT ( 'NONE', #16258 ) ;
#9378=DIRECTION ( 'NONE',  ( 0.000000000000000000, -0.000000000000000000, -1.000000000000000000 ) ) ;
#9417=EDGE_CURVE ( 'NONE', #7634, #15263, #13469, .T. ) ;
#9424=CIRCLE ( 'NONE', #2854, 7.500000000000003553 ) ;
#9442=DIRECTION ( 'NONE',  ( 1.000000000000000000, 0.000000000000000000, 0.000000000000000000 ) ) ;
#9468=AXIS2_PLACEMENT_3D ( 'NONE', #15230, #22561, #20631 ) ;
#9473=CARTESIAN_POINT ( 'NONE',  ( 0.000000000000000000, 0.000000000000000000, 0.000000000000000000 ) ) ;
#9474=ORIENTED_EDGE ( 'NONE', *, *, #18029, .T. ) ;
#9480=ADVANCED_FACE ( 'NONE', ( #16960 ), #6076, .T. ) ;
#9482=LINE ( 'NONE', #5963, #4486 ) ;
#9501=DIRECTION ( 'NONE',  ( 1.000000000000000000, 0.000000000000000000, 0.000000000000000000 ) ) ;
#9506=CYLINDRICAL_SURFACE ( 'NONE', #19559, 35.00000000000000711 ) ;
#9521=DIRECTION ( 'NONE',  ( 0.000000000000000000, 0.000000000000000000, -1.000000000000000000 ) ) ;
#9537=CARTESIAN_POINT ( 'NONE',  ( -117.3074641843675749, 85.22886158240835641, 90.00000000000000000 ) ) ;
#9538=ORIENTED_EDGE ( 'NONE', *, *, #17240, .T. ) ;
#9549=VECTOR ( 'NONE', #23393, 1000.000000000000000 ) ;
#9572=CIRCLE ( 'NONE', #6105, 7.500000000000000000 ) ;
#9577=EDGE_CURVE ( 'NONE', #880, #9666, #10196, .T. ) ;
#9585=DIRECTION ( 'NONE',  ( -0.000000000000000000, -0.000000000000000000, 1.000000000000000000 ) ) ;
#9593=AXIS2_PLACEMENT_3D ( 'NONE', #10083, #1533, #16282 ) ;
#9597=AXIS2_PLACEMENT_3D ( 'NONE', #15977, #21752, #23202 ) ;
#9599=FACE_OUTER_BOUND ( 'NONE', #7217, .T. ) ;
#9607=DIRECTION ( 'NONE',  ( 1.000000000000000000, 0.000000000000000000, 0.000000000000000000 ) ) ;
#9608=VERTEX_POINT ( 'NONE', #21047 ) ;
#9611=CARTESIAN_POINT ( 'NONE',  ( -37.30746418436648071, -137.9031948627975908, -90.00000000000000000 ) ) ;
#9614=VECTOR ( 'NONE', #15069, 1000.000000000000000 ) ;
#9626=CARTESIAN_POINT ( 'NONE',  ( 0.000000000000000000, 0.000000000000000000, -90.00000000000000000 ) ) ;
#9647=AXIS2_PLACEMENT_3D ( 'NONE', #10513, #6853, #14135 ) ;
#9662=DIRECTION ( 'NONE',  ( 1.000000000000000000, 0.000000000000000000, -0.000000000000000000 ) ) ;
#9666=VERTEX_POINT ( 'NONE', #12631 ) ;
#9672=ADVANCED_FACE ( 'NONE', ( #4987 ), #16232, .F. ) ;
#9703=CARTESIAN_POINT ( 'NONE',  ( -85.22886158240879695, 117.3074641843673049, 90.00000000000000000 ) ) ;
#9726=VERTEX_POINT ( 'NONE', #10925 ) ;
#9736=DIRECTION ( 'NONE',  ( 0.000000000000000000, 0.000000000000000000, 1.000000000000000000 ) ) ;
#9778=CARTESIAN_POINT ( 'NONE',  ( 7.497491405671719455, 144.8060344827586334, -90.00000000000000000 ) ) ;
#9779=CARTESIAN_POINT ( 'NONE',  ( 121.5574576620405480, -79.04925354955113903, 90.00000000000000000 ) ) ;
#9791=EDGE_CURVE ( 'NONE', #2320, #20139, #8735, .T. ) ;
#9810=CARTESIAN_POINT ( 'NONE',  ( -7.497491405671719455, -144.8060344827586334, -90.00000000000000000 ) ) ;
#9820=EDGE_CURVE ( 'NONE', #12981, #21305, #258, .T. ) ;
#9836=ORIENTED_EDGE ( 'NONE', *, *, #3694, .T. ) ;
#9840=CARTESIAN_POINT ( 'NONE',  ( 0.000000000000000000, 0.000000000000000000, -90.00000000000000000 ) ) ;
#9858=VERTEX_POINT ( 'NONE', #395 ) ;
#9872=VERTEX_POINT ( 'NONE', #20289 ) ;
#9911=CARTESIAN_POINT ( 'NONE',  ( 85.22886158240964960, -117.3074641843666370, -90.00000000000000000 ) ) ;
#9929=EDGE_CURVE ( 'NONE', #1131, #15709, #6989, .T. ) ;
#9935=EDGE_CURVE ( 'NONE', #4937, #6640, #12736, .T. ) ;
#9938=ORIENTED_EDGE ( 'NONE', *, *, #19363, .T. ) ;
#9939=DIRECTION ( 'NONE',  ( 0.000000000000000000, 0.000000000000000000, 1.000000000000000000 ) ) ;
#9943=CARTESIAN_POINT ( 'NONE',  ( 117.3074641843663386, 85.22886158241004750, -90.00000000000000000 ) ) ;
#9944=AXIS2_PLACEMENT_3D ( 'NONE', #19294, #16160, #19649 ) ;
#9954=DIRECTION ( 'NONE',  ( 1.000000000000000000, 0.000000000000000000, 0.000000000000000000 ) ) ;
#9983=DIRECTION ( 'NONE',  ( 0.000000000000000000, 0.000000000000000000, 1.000000000000000000 ) ) ;
#9993=DIRECTION ( 'NONE',  ( 1.000000000000000000, 0.000000000000000000, 0.000000000000000000 ) ) ;
#9998=CARTESIAN_POINT ( 'NONE',  ( -44.80746418436648071, -137.9031948627975908, -90.00000000000000000 ) ) ;
#10017=CARTESIAN_POINT ( 'NONE',  ( 0.000000000000000000, 0.000000000000000000, -90.00000000000000000 ) ) ;
#10018=DIRECTION ( 'NONE',  ( 0.000000000000000000, 0.000000000000000000, 1.000000000000000000 ) ) ;
#10025=ORIENTED_EDGE ( 'NONE', *, *, #6648, .F. ) ;
#10031=AXIS2_PLACEMENT_3D ( 'NONE', #17930, #1149, #21782 ) ;
#10034=AXIS2_PLACEMENT_3D ( 'NONE', #1604, #9346, #18036 ) ;
#10039=CARTESIAN_POINT ( 'NONE',  ( -137.9031948627971076, -44.80746418436799416, -90.00000000000000000 ) ) ;
#10050=ORIENTED_EDGE ( 'NONE', *, *, #23674, .F. ) ;
#10071=CARTESIAN_POINT ( 'NONE',  ( 0.000000000000000000, 0.000000000000000000, -90.00000000000000000 ) ) ;
#10083=CARTESIAN_POINT ( 'NONE',  ( -85.22886158240795851, -117.3074641843678876, 90.00000000000000000 ) ) ;
#10094=CARTESIAN_POINT ( 'NONE',  ( 137.9031948627967950, 44.80746418436894629, -90.00000000000000000 ) ) ;
#10099=CARTESIAN_POINT ( 'NONE',  ( -109.8074641843675749, 85.22886158240835641, -90.00000000000000000 ) ) ;
#10101=ORIENTED_EDGE ( 'NONE', *, *, #22, .T. ) ;
#10102=DIRECTION ( 'NONE',  ( -0.000000000000000000, 0.000000000000000000, -1.000000000000000000 ) ) ;
#10108=ADVANCED_FACE ( 'NONE', ( #14481 ), #5762, .F. ) ;
#10140=CARTESIAN_POINT ( 'NONE',  ( 135.4018704341550574, 51.87806360044960741, -90.00000000000000000 ) ) ;
#10146=ORIENTED_EDGE ( 'NONE', *, *, #14638, .F. ) ;
#10153=EDGE_LOOP ( 'NONE', ( #19544, #18683, #22892, #22766 ) ) ;
#10179=ORIENTED_EDGE ( 'NONE', *, *, #4490, .F. ) ;
#10190=CIRCLE ( 'NONE', #19417, 7.499999999999998224 ) ;
#10196=LINE ( 'NONE', #12051, #16208 ) ;
#10201=ORIENTED_EDGE ( 'NONE', *, *, #13734, .T. ) ;
#10203=CARTESIAN_POINT ( 'NONE',  ( -137.9031948627974486, 44.80746418436699940, 90.00000000000000000 ) ) ;
#10209=VERTEX_POINT ( 'NONE', #20716 ) ;
#10212=DIRECTION ( 'NONE',  ( 0.000000000000000000, 0.000000000000000000, 1.000000000000000000 ) ) ;
#10217=CARTESIAN_POINT ( 'NONE',  ( -135.4018704341554269, -51.87806360044865528, 90.00000000000000000 ) ) ;
#10223=EDGE_CURVE ( 'NONE', #7547, #10771, #4310, .T. ) ;
#10228=CYLINDRICAL_SURFACE ( 'NONE', #1165, 145.0000000000000284 ) ;
#10230=EDGE_LOOP ( 'NONE', ( #14059, #10656, #10276, #17872 ) ) ;
#10247=ORIENTED_EDGE ( 'NONE', *, *, #8935, .T. ) ;
#10252=DIRECTION ( 'NONE',  ( 0.000000000000000000, 0.000000000000000000, 1.000000000000000000 ) ) ;
#10257=CLOSED_SHELL ( 'NONE', ( #10108, #5194, #7657, #1300, #4262, #5214, #20037, #18323, #22532, #16075, #21922, #18041, #15241, #18252, #8585, #21111, #13905, #4548, #20429, #15090, #7074, #22038, #12808, #8745, #9480, #23751, #15142, #19893, #14465, #2663, #18500, #5462, #10318, #10263, #23026, #23300, #15184, #22878, #21681, #8358, #17281, #3331, #1977, #4075, #15415, #16429, #4790, #12030, #16980, #22445, #9290, #11245, #427, #13163, #9672, #13972, #7370, #15855, #4115, #9109, #18355, #14508, #22752 ) ) ;
#10260=FACE_OUTER_BOUND ( 'NONE', #22577, .T. ) ;
#10263=ADVANCED_FACE ( 'NONE', ( #18652, #8184 ), #15193, .F. ) ;
#10276=ORIENTED_EDGE ( 'NONE', *, *, #2208, .T. ) ;
#10278=DIRECTION ( 'NONE',  ( 0.000000000000000000, 0.000000000000000000, 1.000000000000000000 ) ) ;
#10294=ORIENTED_EDGE ( 'NONE', *, *, #18856, .F. ) ;
#10297=CARTESIAN_POINT ( 'NONE',  ( 121.5574576620388143, 79.04925354955381067, -2.775557561562891351E-14 ) ) ;
#10315=EDGE_CURVE ( 'NONE', #8126, #5651, #22371, .T. ) ;
#10318=ADVANCED_FACE ( 'NONE', ( #11590 ), #4048, .T. ) ;
#10322=EDGE_LOOP ( 'NONE', ( #7505, #857, #13176, #2844 ) ) ;
#10325=CARTESIAN_POINT ( 'NONE',  ( 145.0000000000000284, 1.518794382396763073E-12, 90.00000000000000000 ) ) ;
#10329=ORIENTED_EDGE ( 'NONE', *, *, #4569, .T. ) ;
#10333=DIRECTION ( 'NONE',  ( 1.000000000000000000, 0.000000000000000000, 0.000000000000000000 ) ) ;
#10338=CARTESIAN_POINT ( 'NONE',  ( -117.3074641843669781, -85.22886158240918064, -90.00000000000000000 ) ) ;
#10342=CARTESIAN_POINT ( 'NONE',  ( -117.3074641843675749, 85.22886158240835641, -90.00000000000000000 ) ) ;
#10365=AXIS2_PLACEMENT_3D ( 'NONE', #976, #8356, #6551 ) ;
#10366=CIRCLE ( 'NONE', #15378, 145.0000000000000284 ) ;
#10379=CARTESIAN_POINT ( 'NONE',  ( -144.8060344827586050, -7.497491405672224829, 90.00000000000000000 ) ) ;
#10389=CIRCLE ( 'NONE', #19606, 145.0000000000000284 ) ;
#10392=CIRCLE ( 'NONE', #9597, 145.0000000000000284 ) ;
#10398=CARTESIAN_POINT ( 'NONE',  ( -85.22886158240795851, -117.3074641843678876, -90.00000000000000000 ) ) ;
#10400=EDGE_LOOP ( 'NONE', ( #5841, #6840, #19538, #19999 ) ) ;
#10404=CIRCLE ( 'NONE', #16188, 7.500000000000003553 ) ;
#10415=EDGE_LOOP ( 'NONE', ( #15618, #19365, #13680, #9474 ) ) ;
#10419=VECTOR ( 'NONE', #155, 1000.000000000000000 ) ;
#10431=AXIS2_PLACEMENT_3D ( 'NONE', #6739, #21464, #4927 ) ;
#10449=AXIS2_PLACEMENT_3D ( 'NONE', #11678, #15159, #18872 ) ;
#10451=ORIENTED_EDGE ( 'NONE', *, *, #6601, .T. ) ;
#10454=DIRECTION ( 'NONE',  ( 1.000000000000000000, 0.000000000000000000, 0.000000000000000000 ) ) ;
#10465=EDGE_CURVE ( 'NONE', #3693, #15263, #14630, .T. ) ;
#10474=CARTESIAN_POINT ( 'NONE',  ( -79.04925354955248906, 121.5574576620396812, 90.00000000000000000 ) ) ;
#10475=EDGE_CURVE ( 'NONE', #6640, #9371, #8292, .T. ) ;
#10483=FACE_OUTER_BOUND ( 'NONE', #158, .T. ) ;
#10493=VERTEX_POINT ( 'NONE', #15668 ) ;
#10497=CARTESIAN_POINT ( 'NONE',  ( 160.0000000000000000, 1.959434878635765210E-14, -100.0000000000000000 ) ) ;
#10504=DIRECTION ( 'NONE',  ( 0.3090169943749441761, 0.9510565162951546414, 0.000000000000000000 ) ) ;
#10505=CYLINDRICAL_SURFACE ( 'NONE', #17133, 145.0000000000000284 ) ;
#10513=CARTESIAN_POINT ( 'NONE',  ( 137.9031948627977044, -44.80746418436605438, -90.00000000000000000 ) ) ;
#10526=VERTEX_POINT ( 'NONE', #22028 ) ;
#10527=CARTESIAN_POINT ( 'NONE',  ( 0.000000000000000000, 0.000000000000000000, -90.00000000000000000 ) ) ;
#10532=VECTOR ( 'NONE', #18917, 1000.000000000000000 ) ;
#10547=VERTEX_POINT ( 'NONE', #20100 ) ;
#10556=AXIS2_PLACEMENT_3D ( 'NONE', #1908, #19913, #1570 ) ;
#10576=DIRECTION ( 'NONE',  ( 1.000000000000000000, 0.000000000000000000, 0.000000000000000000 ) ) ;
#10580=ORIENTED_EDGE ( 'NONE', *, *, #6239, .T. ) ;
#10585=LINE ( 'NONE', #13987, #3421 ) ;
#10595=DIRECTION ( 'NONE',  ( -0.000000000000000000, -0.000000000000000000, 1.000000000000000000 ) ) ;
#10621=CARTESIAN_POINT ( 'NONE',  ( 0.000000000000000000, 0.000000000000000000, 90.00000000000000000 ) ) ;
#10645=DIRECTION ( 'NONE',  ( 0.8090169943749468962, 0.5877852522924740253, 0.000000000000000000 ) ) ;
#10651=DIRECTION ( 'NONE',  ( 1.000000000000000000, 0.000000000000000000, 0.000000000000000000 ) ) ;
#10656=ORIENTED_EDGE ( 'NONE', *, *, #14684, .T. ) ;
#10684=ORIENTED_EDGE ( 'NONE', *, *, #1762, .F. ) ;
#10704=CARTESIAN_POINT ( 'NONE',  ( 0.000000000000000000, 0.000000000000000000, 100.0000000000000000 ) ) ;
#10709=CARTESIAN_POINT ( 'NONE',  ( 112.7436279071518754, 91.18044947429078206, -2.775557561562891351E-14 ) ) ;
#10720=AXIS2_PLACEMENT_3D ( 'NONE', #23638, #8806, #14142 ) ;
#10747=DIRECTION ( 'NONE',  ( 0.000000000000000000, 0.000000000000000000, -1.000000000000000000 ) ) ;
#10760=DIRECTION ( 'NONE',  ( 0.8090169943749468962, 0.5877852522924740253, 0.000000000000000000 ) ) ;
#10770=STYLED_ITEM('',(#23913),#19817);
#10771=VERTEX_POINT ( 'NONE', #17541 ) ;
#10777=CIRCLE ( 'NONE', #16539, 145.0000000000000284 ) ;
#10788=VECTOR ( 'NONE', #23597, 1000.000000000000000 ) ;
#10789=FACE_OUTER_BOUND ( 'NONE', #21465, .T. ) ;
#10803=VECTOR ( 'NONE', #9585, 1000.000000000000000 ) ;
#10808=DIRECTION ( 'NONE',  ( 0.000000000000000000, -0.000000000000000000, 1.000000000000000000 ) ) ;
#10842=ORIENTED_EDGE ( 'NONE', *, *, #8034, .F. ) ;
#10844=EDGE_CURVE ( 'NONE', #18342, #8126, #724, .T. ) ;
#10892=DIRECTION ( 'NONE',  ( 0.000000000000000000, 0.000000000000000000, 1.000000000000000000 ) ) ;
#10918=FACE_OUTER_BOUND ( 'NONE', #461, .T. ) ;
#10920=CARTESIAN_POINT ( 'NONE',  ( 140.0355749532205891, 37.61698748598766429, -90.00000000000000000 ) ) ;
#10925=CARTESIAN_POINT ( 'NONE',  ( 144.8060344827585482, 7.497491405673236464, 90.00000000000000000 ) ) ;
#10931=VERTEX_POINT ( 'NONE', #4229 ) ;
#10948=( NAMED_UNIT ( * ) PLANE_ANGLE_UNIT ( ) SI_UNIT ( $, .RADIAN. ) );
#10970=EDGE_CURVE ( 'NONE', #18161, #7547, #16387, .T. ) ;
#10972=( LENGTH_UNIT ( ) NAMED_UNIT ( * ) SI_UNIT ( .MILLI., .METRE. ) );
#10981=VERTEX_POINT ( 'NONE', #18753 ) ;
#10983=ORIENTED_EDGE ( 'NONE', *, *, #23208, .F. ) ;
#10994=CARTESIAN_POINT ( 'NONE',  ( 135.4018704341561374, -51.87806360044677234, -90.00000000000000000 ) ) ;
#11008=CARTESIAN_POINT ( 'NONE',  ( 0.000000000000000000, 0.000000000000000000, 90.00000000000000000 ) ) ;
#11016=EDGE_CURVE ( 'NONE', #17622, #9308, #2716, .T. ) ;
#11029=AXIS2_PLACEMENT_3D ( 'NONE', #8130, #17416, #23062 ) ;
#11044=VERTEX_POINT ( 'NONE', #15409 ) ;
#11046=CIRCLE ( 'NONE', #22964, 7.500000000000000888 ) ;
#11050=DIRECTION ( 'NONE',  ( 0.000000000000000000, 0.000000000000000000, 1.000000000000000000 ) ) ;
#11076=CYLINDRICAL_SURFACE ( 'NONE', #4166, 7.500000000000007105 ) ;
#11081=VERTEX_POINT ( 'NONE', #2461 ) ;
#11084=ORIENTED_EDGE ( 'NONE', *, *, #2032, .F. ) ;
#11097=CIRCLE ( 'NONE', #20711, 7.500000000000001776 ) ;
#11120=AXIS2_PLACEMENT_3D ( 'NONE', #1040, #8424, #3326 ) ;
#11121=VERTEX_POINT ( 'NONE', #15171 ) ;
#11136=DIRECTION ( 'NONE',  ( 0.000000000000000000, 0.000000000000000000, 1.000000000000000000 ) ) ;
#11142=EDGE_CURVE ( 'NONE', #13673, #11044, #13740, .T. ) ;
#11177=CARTESIAN_POINT ( 'NONE',  ( 0.000000000000000000, 0.000000000000000000, -90.00000000000000000 ) ) ;
#11199=DIRECTION ( 'NONE',  ( 1.000000000000000000, 0.000000000000000000, 0.000000000000000000 ) ) ;
#11210=AXIS2_PLACEMENT_3D ( 'NONE', #9473, #14914, #3769 ) ;
#11213=AXIS2_PLACEMENT_3D ( 'NONE', #4786, #23722, #6965 ) ;
#11216=CARTESIAN_POINT ( 'NONE',  ( -145.0000000000000284, -5.062647941322544249E-13, -90.00000000000000000 ) ) ;
#11218=DIRECTION ( 'NONE',  ( 0.000000000000000000, 0.000000000000000000, -1.000000000000000000 ) ) ;
#11245=ADVANCED_FACE ( 'NONE', ( #1001 ), #19721, .F. ) ;
#11268=CARTESIAN_POINT ( 'NONE',  ( -137.5000000000000000, -5.062647941322544249E-13, -90.00000000000000000 ) ) ;
#11295=EDGE_LOOP ( 'NONE', ( #23602, #10842, #7625, #20386 ) ) ;
#11303=VERTEX_POINT ( 'NONE', #21535 ) ;
#11313=DIRECTION ( 'NONE',  ( 0.000000000000000000, 0.000000000000000000, 1.000000000000000000 ) ) ;
#11369=ORIENTED_EDGE ( 'NONE', *, *, #8740, .F. ) ;
#11387=CARTESIAN_POINT ( 'NONE',  ( -112.7436279071525433, -91.18044947428992941, -2.775557561562891351E-14 ) ) ;
#11388=DIRECTION ( 'NONE',  ( 0.000000000000000000, 0.000000000000000000, 1.000000000000000000 ) ) ;
#11397=CARTESIAN_POINT ( 'NONE',  ( 91.18044947429038416, -112.7436279071521881, -2.775557561562891351E-14 ) ) ;
#11446=CYLINDRICAL_SURFACE ( 'NONE', #15411, 145.0000000000000284 ) ;
#11450=DIRECTION ( 'NONE',  ( -0.5877852522924773560, 0.8090169943749444537, 0.000000000000000000 ) ) ;
#11464=CIRCLE ( 'NONE', #2159, 7.500000000000004441 ) ;
#11466=CARTESIAN_POINT ( 'NONE',  ( 0.000000000000000000, 0.000000000000000000, -90.00000000000000000 ) ) ;
#11469=DIRECTION ( 'NONE',  ( 1.000000000000000000, 0.000000000000000000, 0.000000000000000000 ) ) ;
#11470=CARTESIAN_POINT ( 'NONE',  ( 44.80746418436557832, 137.9031948627978750, 90.00000000000000000 ) ) ;
#11505=AXIS2_PLACEMENT_3D ( 'NONE', #701, #17258, #11738 ) ;
#11512=AXIS2_PLACEMENT_3D ( 'NONE', #4280, #18992, #5965 ) ;
#11514=EDGE_CURVE ( 'NONE', #17056, #10547, #2644, .T. ) ;
#11532=CYLINDRICAL_SURFACE ( 'NONE', #15287, 35.00000000000000711 ) ;
#11533=ORIENTED_EDGE ( 'NONE', *, *, #12332, .T. ) ;
#11549=DIRECTION ( 'NONE',  ( -0.8090169943749507819, 0.5877852522924686962, 0.000000000000000000 ) ) ;
#11575=FACE_OUTER_BOUND ( 'NONE', #17087, .T. ) ;
#11581=CARTESIAN_POINT ( 'NONE',  ( -117.3074641843669781, -85.22886158240918064, 90.00000000000000000 ) ) ;
#11590=FACE_OUTER_BOUND ( 'NONE', #12019, .T. ) ;
#11594=VECTOR ( 'NONE', #15536, 1000.000000000000000 ) ;
#11602=DIRECTION ( 'NONE',  ( 0.000000000000000000, 0.000000000000000000, 1.000000000000000000 ) ) ;
#11606=EDGE_LOOP ( 'NONE', ( #4807, #1480 ) ) ;
#11671=ORIENTED_EDGE ( 'NONE', *, *, #19929, .T. ) ;
#11678=CARTESIAN_POINT ( 'NONE',  ( 44.80746418436846312, -137.9031948627969655, 90.00000000000000000 ) ) ;
#11684=CARTESIAN_POINT ( 'NONE',  ( -44.80746418436748968, 137.9031948627972781, -90.00000000000000000 ) ) ;
#11687=EDGE_CURVE ( 'NONE', #4754, #2497, #16060, .T. ) ;
#11695=DIRECTION ( 'NONE',  ( 0.8090169943749552228, -0.5877852522924623679, 0.000000000000000000 ) ) ;
#11696=VERTEX_POINT ( 'NONE', #3130 ) ;
#11701=FACE_OUTER_BOUND ( 'NONE', #8732, .T. ) ;
#11719=EDGE_CURVE ( 'NONE', #13438, #2480, #8633, .T. ) ;
#11723=EDGE_CURVE ( 'NONE', #17692, #13438, #10190, .T. ) ;
#11733=DIRECTION ( 'NONE',  ( -0.5877852522924773560, 0.8090169943749444537, 0.000000000000000000 ) ) ;
#11736=VERTEX_POINT ( 'NONE', #6999 ) ;
#11738=DIRECTION ( 'NONE',  ( 1.000000000000000000, 0.000000000000000000, 0.000000000000000000 ) ) ;
#11739=CARTESIAN_POINT ( 'NONE',  ( -117.3074641843669781, -85.22886158240918064, -90.00000000000000000 ) ) ;
#11746=ORIENTED_EDGE ( 'NONE', *, *, #16496, .T. ) ;
#11761=ORIENTED_EDGE ( 'NONE', *, *, #20454, .F. ) ;
#11764=VERTEX_POINT ( 'NONE', #14387 ) ;
#11782=CARTESIAN_POINT ( 'NONE',  ( -37.61698748598514896, -140.0355749532212428, -90.00000000000000000 ) ) ;
#11795=DIRECTION ( 'NONE',  ( -1.000000000000000000, 0.000000000000000000, 0.000000000000000000 ) ) ;
#11801=DIRECTION ( 'NONE',  ( 1.000000000000000000, 0.000000000000000000, 0.000000000000000000 ) ) ;
#11805=VERTEX_POINT ( 'NONE', #7107 ) ;
#11806=CIRCLE ( 'NONE', #6771, 7.499999999999996447 ) ;
#11810=CARTESIAN_POINT ( 'NONE',  ( 0.000000000000000000, 0.000000000000000000, 90.00000000000000000 ) ) ;
#11815=DIRECTION ( 'NONE',  ( 0.000000000000000000, 0.000000000000000000, 1.000000000000000000 ) ) ;
#11833=CIRCLE ( 'NONE', #7535, 160.0000000000000000 ) ;
#11856=ORIENTED_EDGE ( 'NONE', *, *, #23674, .T. ) ;
#11889=EDGE_LOOP ( 'NONE', ( #10179, #9121, #23239, #1571 ) ) ;
#11899=DIRECTION ( 'NONE',  ( 1.000000000000000000, 0.000000000000000000, 0.000000000000000000 ) ) ;
#11911=VERTEX_POINT ( 'NONE', #2013 ) ;
#11924=CIRCLE ( 'NONE', #4959, 145.0000000000000284 ) ;
#11926=ADVANCED_BREP_SHAPE_REPRESENTATION ( '', ( #19817, #11210 ), #17342 ) ;
#11960=CIRCLE ( 'NONE', #6892, 7.500000000000000000 ) ;
#11962=DIRECTION ( 'NONE',  ( 0.000000000000000000, 0.000000000000000000, 1.000000000000000000 ) ) ;
#11974=CARTESIAN_POINT ( 'NONE',  ( 117.3074641843682144, -85.22886158240748955, -90.00000000000000000 ) ) ;
#11983=ORIENTED_EDGE ( 'NONE', *, *, #15374, .F. ) ;
#11987=CARTESIAN_POINT ( 'NONE',  ( 144.8060344827587471, -7.497491405670203335, -2.775557561562891351E-14 ) ) ;
#12003=DIRECTION ( 'NONE',  ( -0.000000000000000000, -0.000000000000000000, 1.000000000000000000 ) ) ;
#12007=ORIENTED_EDGE ( 'NONE', *, *, #13051, .F. ) ;
#12019=EDGE_LOOP ( 'NONE', ( #19316, #5992, #8962, #21742 ) ) ;
#12030=ADVANCED_FACE ( 'NONE', ( #21094 ), #19280, .F. ) ;
#12036=DIRECTION ( 'NONE',  ( -0.000000000000000000, -0.000000000000000000, 1.000000000000000000 ) ) ;
#12051=CARTESIAN_POINT ( 'NONE',  ( -109.8074641843669781, -85.22886158240918064, -90.00000000000000000 ) ) ;
#12059=EDGE_CURVE ( 'NONE', #7634, #21672, #9424, .T. ) ;
#12065=ORIENTED_EDGE ( 'NONE', *, *, #17834, .T. ) ;
#12073=DIRECTION ( 'NONE',  ( 0.000000000000000000, 0.000000000000000000, 1.000000000000000000 ) ) ;
#12074=EDGE_CURVE ( 'NONE', #20363, #21672, #16032, .T. ) ;
#12083=ORIENTED_EDGE ( 'NONE', *, *, #20234, .F. ) ;
#12113=ORIENTED_EDGE ( 'NONE', *, *, #4490, .T. ) ;
#12114=CARTESIAN_POINT ( 'NONE',  ( 37.61698748598716691, -140.0355749532207028, 90.00000000000000000 ) ) ;
#12120=CARTESIAN_POINT ( 'NONE',  ( -37.30746418436748968, 137.9031948627972781, -90.00000000000000000 ) ) ;
#12131=ORIENTED_EDGE ( 'NONE', *, *, #2636, .F. ) ;
#12133=DIRECTION ( 'NONE',  ( -0.000000000000000000, -0.000000000000000000, 1.000000000000000000 ) ) ;
#12156=CARTESIAN_POINT ( 'NONE',  ( -135.4018704341557964, 51.87806360044768894, 90.00000000000000000 ) ) ;
#12195=EDGE_CURVE ( 'NONE', #9608, #9858, #78, .T. ) ;
#12200=ORIENTED_EDGE ( 'NONE', *, *, #21284, .F. ) ;
#12203=VECTOR ( 'NONE', #19150, 1000.000000000000000 ) ;
#12215=ORIENTED_EDGE ( 'NONE', *, *, #8405, .T. ) ;
#12216=ORIENTED_EDGE ( 'NONE', *, *, #19085, .T. ) ;
#12218=LINE ( 'NONE', #11987, #3446 ) ;
#12221=AXIS2_PLACEMENT_3D ( 'NONE', #11216, #3912, #548 ) ;
#12239=CARTESIAN_POINT ( 'NONE',  ( -91.18044947428954572, 112.7436279071528844, -2.775557561562891351E-14 ) ) ;
#12263=DIRECTION ( 'NONE',  ( -0.5877852522924643663, -0.8090169943749537795, 0.000000000000000000 ) ) ;
#12288=CARTESIAN_POINT ( 'NONE',  ( 51.87806360044913134, -135.4018704341552564, 90.00000000000000000 ) ) ;
#12292=DIRECTION ( 'NONE',  ( 1.000000000000000000, 0.000000000000000000, 0.000000000000000000 ) ) ;
#12332=EDGE_CURVE ( 'NONE', #3110, #10547, #19793, .T. ) ;
#12334=DIRECTION ( 'NONE',  ( 1.000000000000000000, 0.000000000000000000, -0.000000000000000000 ) ) ;
#12347=FACE_OUTER_BOUND ( 'NONE', #11295, .T. ) ;
#12352=VECTOR ( 'NONE', #7888, 1000.000000000000000 ) ;
#12357=FACE_OUTER_BOUND ( 'NONE', #8798, .T. ) ;
#12358=DIRECTION ( 'NONE',  ( 0.000000000000000000, -0.000000000000000000, 1.000000000000000000 ) ) ;
#12359=EDGE_LOOP ( 'NONE', ( #18032, #5942, #14545, #3187 ) ) ;
#12407=VERTEX_POINT ( 'NONE', #5242 ) ;
#12429=DIRECTION ( 'NONE',  ( -0.000000000000000000, 1.000000000000000000, 0.000000000000000000 ) ) ;
#12433=ORIENTED_EDGE ( 'NONE', *, *, #17174, .F. ) ;
#12489=DIRECTION ( 'NONE',  ( 0.000000000000000000, 0.000000000000000000, 1.000000000000000000 ) ) ;
#12498=ORIENTED_EDGE ( 'NONE', *, *, #20501, .F. ) ;
#12539=CARTESIAN_POINT ( 'NONE',  ( 0.000000000000000000, 0.000000000000000000, 90.00000000000000000 ) ) ;
#12549=DIRECTION ( 'NONE',  ( 0.000000000000000000, 0.000000000000000000, -1.000000000000000000 ) ) ;
#12550=AXIS2_PLACEMENT_3D ( 'NONE', #11974, #2747, #8304 ) ;
#12558=EDGE_CURVE ( 'NONE', #21317, #19753, #16341, .T. ) ;
#12572=VERTEX_POINT ( 'NONE', #11782 ) ;
#12574=ORIENTED_EDGE ( 'NONE', *, *, #12195, .T. ) ;
#12612=DIRECTION ( 'NONE',  ( 0.000000000000000000, -0.000000000000000000, -1.000000000000000000 ) ) ;
#12625=FACE_OUTER_BOUND ( 'NONE', #22194, .T. ) ;
#12631=CARTESIAN_POINT ( 'NONE',  ( -109.8074641843669781, -85.22886158240918064, 90.00000000000000000 ) ) ;
#12637=AXIS2_PLACEMENT_3D ( 'NONE', #21569, #17944, #8775 ) ;
#12650=CYLINDRICAL_SURFACE ( 'NONE', #8440, 7.500000000000007105 ) ;
#12676=DIRECTION ( 'NONE',  ( 0.9510565162951534202, 0.3090169943749478398, 0.000000000000000000 ) ) ;
#12696=DIRECTION ( 'NONE',  ( 1.000000000000000000, 0.000000000000000000, 0.000000000000000000 ) ) ;
#12705=EDGE_CURVE ( 'NONE', #9872, #7615, #7975, .T. ) ;
#12707=ORIENTED_EDGE ( 'NONE', *, *, #14734, .T. ) ;
#12711=ORIENTED_EDGE ( 'NONE', *, *, #22169, .F. ) ;
#12715=PLANE ( 'NONE',  #14241 ) ;
#12736=CIRCLE ( 'NONE', #3859, 145.0000000000000284 ) ;
#12781=MECHANICAL_DESIGN_GEOMETRIC_PRESENTATION_REPRESENTATION('',(#14675),#20420);
#12786=LINE ( 'NONE', #16466, #3401 ) ;
#12790=AXIS2_PLACEMENT_3D ( 'NONE', #11470, #2252, #467 ) ;
#12808=ADVANCED_FACE ( 'NONE', ( #1406 ), #10505, .T. ) ;
#12835=ORIENTED_EDGE ( 'NONE', *, *, #15383, .T. ) ;
#12836=EDGE_LOOP ( 'NONE', ( #5481, #4522, #14606, #20538 ) ) ;
#12843=ORIENTED_EDGE ( 'NONE', *, *, #6648, .T. ) ;
#12848=ORIENTED_EDGE ( 'NONE', *, *, #14524, .F. ) ;
#12883=ORIENTED_EDGE ( 'NONE', *, *, #9935, .F. ) ;
#12886=CARTESIAN_POINT ( 'NONE',  ( -85.22886158240795851, -117.3074641843678876, -90.00000000000000000 ) ) ;
#12892=ORIENTED_EDGE ( 'NONE', *, *, #16478, .T. ) ;
#12932=CIRCLE ( 'NONE', #22183, 7.500000000000000000 ) ;
#12962=CARTESIAN_POINT ( 'NONE',  ( 0.000000000000000000, 0.000000000000000000, 100.0000000000000000 ) ) ;
#12972=APPLICATION_CONTEXT ( 'automotive_design' ) ;
#12981=VERTEX_POINT ( 'NONE', #20336 ) ;
#12989=ORIENTED_EDGE ( 'NONE', *, *, #7650, .T. ) ;
#12993=ORIENTED_EDGE ( 'NONE', *, *, #5924, .F. ) ;
#13003=DIRECTION ( 'NONE',  ( 1.000000000000000000, 0.000000000000000000, 0.000000000000000000 ) ) ;
#13008=ORIENTED_EDGE ( 'NONE', *, *, #15383, .F. ) ;
#13012=ORIENTED_EDGE ( 'NONE', *, *, #21253, .F. ) ;
#13051=EDGE_CURVE ( 'NONE', #14252, #20139, #915, .T. ) ;
#13058=EDGE_CURVE ( 'NONE', #3015, #19875, #14441, .T. ) ;
#13067=EDGE_CURVE ( 'NONE', #2497, #17622, #22526, .T. ) ;
#13068=EDGE_CURVE ( 'NONE', #22784, #17056, #14088, .T. ) ;
#13072=VERTEX_POINT ( 'NONE', #10217 ) ;
#13077=EDGE_LOOP ( 'NONE', ( #8030, #2406 ) ) ;
#13097=AXIS2_PLACEMENT_3D ( 'NONE', #2370, #2239, #8185 ) ;
#13108=ORIENTED_EDGE ( 'NONE', *, *, #19832, .T. ) ;
#13109=CIRCLE ( 'NONE', #20778, 160.0000000000000000 ) ;
#13114=VECTOR ( 'NONE', #10747, 1000.000000000000000 ) ;
#13127=DIRECTION ( 'NONE',  ( -0.000000000000000000, -0.000000000000000000, -1.000000000000000000 ) ) ;
#13131=AXIS2_PLACEMENT_3D ( 'NONE', #18605, #11050, #5701 ) ;
#13163=ADVANCED_FACE ( 'NONE', ( #11701 ), #20841, .F. ) ;
#13176=ORIENTED_EDGE ( 'NONE', *, *, #116, .T. ) ;
#13199=VERTEX_POINT ( 'NONE', #8042 ) ;
#13207=DIRECTION ( 'NONE',  ( 0.000000000000000000, 0.000000000000000000, 1.000000000000000000 ) ) ;
#13226=EDGE_LOOP ( 'NONE', ( #6287, #17828, #17651, #17608 ) ) ;
#13263=CARTESIAN_POINT ( 'NONE',  ( 0.000000000000000000, 0.000000000000000000, -100.0000000000000000 ) ) ;
#13268=ORIENTED_EDGE ( 'NONE', *, *, #5917, .T. ) ;
#13309=DIRECTION ( 'NONE',  ( 0.000000000000000000, -0.000000000000000000, 1.000000000000000000 ) ) ;
#13320=VERTEX_POINT ( 'NONE', #3299 ) ;
#13321=VERTEX_POINT ( 'NONE', #17813 ) ;
#13342=ORIENTED_EDGE ( 'NONE', *, *, #1307, .F. ) ;
#13349=AXIS2_PLACEMENT_3D ( 'NONE', #1091, #22830, #17296 ) ;
#13378=ORIENTED_EDGE ( 'NONE', *, *, #10465, .T. ) ;
#13396=EDGE_CURVE ( 'NONE', #18184, #9858, #1317, .T. ) ;
#13400=ORIENTED_EDGE ( 'NONE', *, *, #22, .F. ) ;
#13402=CARTESIAN_POINT ( 'NONE',  ( 0.000000000000000000, 0.000000000000000000, -100.0000000000000000 ) ) ;
#13411=FACE_OUTER_BOUND ( 'NONE', #16900, .T. ) ;
#13414=ORIENTED_EDGE ( 'NONE', *, *, #9929, .F. ) ;
#13438=VERTEX_POINT ( 'NONE', #22486 ) ;
#13452=CARTESIAN_POINT ( 'NONE',  ( -145.0000000000000284, -5.062647941322544249E-13, -90.00000000000000000 ) ) ;
#13459=AXIS2_PLACEMENT_3D ( 'NONE', #8524, #16121, #14338 ) ;
#13461=VERTEX_POINT ( 'NONE', #2080 ) ;
#13468=CARTESIAN_POINT ( 'NONE',  ( -109.8074641843669781, -85.22886158240918064, -90.00000000000000000 ) ) ;
#13469=CIRCLE ( 'NONE', #6100, 145.0000000000000284 ) ;
#13474=CARTESIAN_POINT ( 'NONE',  ( 51.87806360044912424, -135.4018704341552279, -2.775557561562891351E-14 ) ) ;
#13480=CARTESIAN_POINT ( 'NONE',  ( 0.000000000000000000, 0.000000000000000000, -100.0000000000000000 ) ) ;
#13485=CARTESIAN_POINT ( 'NONE',  ( 7.499999999999999112, 41.99999999999998579, 100.0000000000000000 ) ) ;
#13489=ORIENTED_EDGE ( 'NONE', *, *, #20501, .T. ) ;
#13502=VERTEX_POINT ( 'NONE', #13485 ) ;
#13516=VECTOR ( 'NONE', #12429, 1000.000000000000000 ) ;
#13526=DIRECTION ( 'NONE',  ( 0.5877852522924719159, 0.8090169943749482284, 0.000000000000000000 ) ) ;
#13533=ORIENTED_EDGE ( 'NONE', *, *, #18176, .F. ) ;
#13547=EDGE_CURVE ( 'NONE', #18184, #8675, #8443, .T. ) ;
#13576=DIRECTION ( 'NONE',  ( 1.000000000000000000, 0.000000000000000000, 0.000000000000000000 ) ) ;
#13587=CYLINDRICAL_SURFACE ( 'NONE', #7292, 7.500000000000007105 ) ;
#13598=CARTESIAN_POINT ( 'NONE',  ( 0.000000000000000000, 0.000000000000000000, 100.0000000000000000 ) ) ;
#13607=EDGE_CURVE ( 'NONE', #11805, #19135, #17310, .T. ) ;
#13608=CARTESIAN_POINT ( 'NONE',  ( 79.04925354955072692, 121.5574576620408322, -2.775557561562891351E-14 ) ) ;
#13621=CARTESIAN_POINT ( 'NONE',  ( -51.87806360044718446, -135.4018704341559953, 90.00000000000000000 ) ) ;
#13640=CARTESIAN_POINT ( 'NONE',  ( -135.4018704341554269, -51.87806360044866238, -2.775557561562891351E-14 ) ) ;
#13650=ORIENTED_EDGE ( 'NONE', *, *, #2777, .F. ) ;
#13664=VERTEX_POINT ( 'NONE', #13719 ) ;
#13673=VERTEX_POINT ( 'NONE', #6906 ) ;
#13676=CYLINDRICAL_SURFACE ( 'NONE', #9076, 7.500000000000007105 ) ;
#13680=ORIENTED_EDGE ( 'NONE', *, *, #7243, .T. ) ;
#13692=CARTESIAN_POINT ( 'NONE',  ( -91.18044947428876412, -112.7436279071535239, 90.00000000000000000 ) ) ;
#13694=DIRECTION ( 'NONE',  ( 0.000000000000000000, -0.000000000000000000, 1.000000000000000000 ) ) ;
#13715=AXIS2_PLACEMENT_3D ( 'NONE', #4752, #8511, #15887 ) ;
#13719=CARTESIAN_POINT ( 'NONE',  ( 7.499999999999997335, 34.18698582794336005, -100.0000000000000000 ) ) ;
#13720=EDGE_LOOP ( 'NONE', ( #13400, #23427, #13414, #17853 ) ) ;
#13729=CARTESIAN_POINT ( 'NONE',  ( 0.000000000000000000, -145.0000000000000284, -90.00000000000000000 ) ) ;
#13734=EDGE_CURVE ( 'NONE', #20344, #19833, #5347, .T. ) ;
#13740=LINE ( 'NONE', #19240, #18672 ) ;
#13748=DIRECTION ( 'NONE',  ( 0.8090169943749552228, -0.5877852522924623679, 0.000000000000000000 ) ) ;
#13749=FACE_OUTER_BOUND ( 'NONE', #5159, .T. ) ;
#13767=EDGE_CURVE ( 'NONE', #11303, #2646, #10777, .T. ) ;
#13770=DIRECTION ( 'NONE',  ( -0.000000000000000000, -0.000000000000000000, 1.000000000000000000 ) ) ;
#13793=CYLINDRICAL_SURFACE ( 'NONE', #8773, 7.500000000000000000 ) ;
#13798=EDGE_CURVE ( 'NONE', #15856, #3142, #10392, .T. ) ;
#13809=DIRECTION ( 'NONE',  ( 0.000000000000000000, -0.000000000000000000, 1.000000000000000000 ) ) ;
#13813=ORIENTED_EDGE ( 'NONE', *, *, #6361, .F. ) ;
#13826=AXIS2_PLACEMENT_3D ( 'NONE', #21462, #1997, #1876 ) ;
#13837=ORIENTED_EDGE ( 'NONE', *, *, #15248, .T. ) ;
#13839=ORIENTED_EDGE ( 'NONE', *, *, #17174, .T. ) ;
#13853=CIRCLE ( 'NONE', #7632, 35.00000000000000711 ) ;
#13858=ORIENTED_EDGE ( 'NONE', *, *, #11687, .F. ) ;
#13875=ORIENTED_EDGE ( 'NONE', *, *, #1676, .T. ) ;
#13877=CARTESIAN_POINT ( 'NONE',  ( 0.000000000000000000, 0.000000000000000000, -90.00000000000000000 ) ) ;
#13887=CIRCLE ( 'NONE', #22315, 145.0000000000000284 ) ;
#13889=AXIS2_PLACEMENT_3D ( 'NONE', #217, #9161, #20723 ) ;
#13905=ADVANCED_FACE ( 'NONE', ( #10918 ), #2046, .T. ) ;
#13908=VERTEX_POINT ( 'NONE', #9204 ) ;
#13913=DIRECTION ( 'NONE',  ( 0.000000000000000000, 0.000000000000000000, -1.000000000000000000 ) ) ;
#13916=ORIENTED_EDGE ( 'NONE', *, *, #18706, .F. ) ;
#13920=DIRECTION ( 'NONE',  ( 1.000000000000000000, 0.000000000000000000, 0.000000000000000000 ) ) ;
#13921=DIRECTION ( 'NONE',  ( 1.000000000000000000, 0.000000000000000000, 0.000000000000000000 ) ) ;
#13930=ORIENTED_EDGE ( 'NONE', *, *, #14119, .T. ) ;
#13931=VERTEX_POINT ( 'NONE', #18590 ) ;
#13947=AXIS2_PLACEMENT_3D ( 'NONE', #13402, #5874, #20965 ) ;
#13957=DIRECTION ( 'NONE',  ( 0.000000000000000000, 0.000000000000000000, -1.000000000000000000 ) ) ;
#13962=CARTESIAN_POINT ( 'NONE',  ( 0.000000000000000000, 0.000000000000000000, -90.00000000000000000 ) ) ;
#13972=ADVANCED_FACE ( 'NONE', ( #15359 ), #13587, .F. ) ;
#13973=CARTESIAN_POINT ( 'NONE',  ( 160.0000000000000000, 1.959434878635765210E-14, 90.00000000000000000 ) ) ;
#13983=CARTESIAN_POINT ( 'NONE',  ( -160.0000000000000000, 0.000000000000000000, 100.0000000000000000 ) ) ;
#13987=CARTESIAN_POINT ( 'NONE',  ( -7.499999999999999112, 41.99999999999998579, -100.0000000000000000 ) ) ;
#13992=DIRECTION ( 'NONE',  ( 0.5877852522924719159, 0.8090169943749482284, 0.000000000000000000 ) ) ;
#14020=LINE ( 'NONE', #16046, #2292 ) ;
#14053=CARTESIAN_POINT ( 'NONE',  ( -7.499999999999997335, 34.18698582794336005, -100.0000000000000000 ) ) ;
#14059=ORIENTED_EDGE ( 'NONE', *, *, #423, .F. ) ;
#14064=LINE ( 'NONE', #13640, #21192 ) ;
#14079=ORIENTED_EDGE ( 'NONE', *, *, #18138, .T. ) ;
#14088=CIRCLE ( 'NONE', #19430, 7.500000000000006217 ) ;
#14095=CYLINDRICAL_SURFACE ( 'NONE', #15751, 7.500000000000000000 ) ;
#14102=CARTESIAN_POINT ( 'NONE',  ( 0.000000000000000000, -145.0000000000000284, -90.00000000000000000 ) ) ;
#14119=EDGE_CURVE ( 'NONE', #18305, #13199, #9243, .T. ) ;
#14132=ORIENTED_EDGE ( 'NONE', *, *, #4432, .T. ) ;
#14135=DIRECTION ( 'NONE',  ( -0.3090169943749370707, -0.9510565162951569729, 0.000000000000000000 ) ) ;
#14142=DIRECTION ( 'NONE',  ( 1.000000000000000000, 0.000000000000000000, 0.000000000000000000 ) ) ;
#14151=ORIENTED_EDGE ( 'NONE', *, *, #2376, .F. ) ;
#14161=DIRECTION ( 'NONE',  ( 0.000000000000000000, 0.000000000000000000, 1.000000000000000000 ) ) ;
#14164=DIRECTION ( 'NONE',  ( -0.000000000000000000, 0.000000000000000000, 1.000000000000000000 ) ) ;
#14187=DIRECTION ( 'NONE',  ( 0.000000000000000000, -0.000000000000000000, 1.000000000000000000 ) ) ;
#14205=VERTEX_POINT ( 'NONE', #1892 ) ;
#14210=CARTESIAN_POINT ( 'NONE',  ( -7.499999999999999112, 0.000000000000000000, -100.0000000000000000 ) ) ;
#14241=AXIS2_PLACEMENT_3D ( 'NONE', #3360, #17869, #23654 ) ;
#14252=VERTEX_POINT ( 'NONE', #7940 ) ;
#14253=DIRECTION ( 'NONE',  ( -0.000000000000000000, -0.000000000000000000, 1.000000000000000000 ) ) ;
#14257=CARTESIAN_POINT ( 'NONE',  ( 0.000000000000000000, 0.000000000000000000, 90.00000000000000000 ) ) ;
#14275=ORIENTED_EDGE ( 'NONE', *, *, #21555, .T. ) ;
#14301=CARTESIAN_POINT ( 'NONE',  ( -135.4018704341554269, -51.87806360044865528, -90.00000000000000000 ) ) ;
#14306=DIRECTION ( 'NONE',  ( 0.000000000000000000, 0.000000000000000000, 1.000000000000000000 ) ) ;
#14338=DIRECTION ( 'NONE',  ( 1.000000000000000000, 0.000000000000000000, 0.000000000000000000 ) ) ;
#14363=ORIENTED_EDGE ( 'NONE', *, *, #17444, .F. ) ;
#14364=CARTESIAN_POINT ( 'NONE',  ( -44.80746418436748968, 137.9031948627972781, -90.00000000000000000 ) ) ;
#14371=DIRECTION ( 'NONE',  ( 0.000000000000000000, 0.000000000000000000, 1.000000000000000000 ) ) ;
#14375=CARTESIAN_POINT ( 'NONE',  ( 44.80746418436846312, -137.9031948627969655, -90.00000000000000000 ) ) ;
#14387=CARTESIAN_POINT ( 'NONE',  ( -51.87806360044816500, 135.4018704341555974, -90.00000000000000000 ) ) ;
#14399=CYLINDRICAL_SURFACE ( 'NONE', #21476, 7.500000000000000888 ) ;
#14405=CYLINDRICAL_SURFACE ( 'NONE', #235, 7.500000000000007105 ) ;
#14417=ORIENTED_EDGE ( 'NONE', *, *, #22626, .T. ) ;
#14437=CARTESIAN_POINT ( 'NONE',  ( -109.8074641843675749, 85.22886158240835641, 90.00000000000000000 ) ) ;
#14438=DIRECTION ( 'NONE',  ( 1.000000000000000000, 0.000000000000000000, 0.000000000000000000 ) ) ;
#14441=CIRCLE ( 'NONE', #3988, 160.0000000000000000 ) ;
#14465=ADVANCED_FACE ( 'NONE', ( #21688 ), #23612, .T. ) ;
#14481=FACE_OUTER_BOUND ( 'NONE', #15636, .T. ) ;
#14487=DIRECTION ( 'NONE',  ( 0.000000000000000000, 0.000000000000000000, 1.000000000000000000 ) ) ;
#14490=CYLINDRICAL_SURFACE ( 'NONE', #1444, 7.500000000000000000 ) ;
#14492=ORIENTED_EDGE ( 'NONE', *, *, #2033, .T. ) ;
#14502=DIRECTION ( 'NONE',  ( -0.000000000000000000, 0.000000000000000000, 1.000000000000000000 ) ) ;
#14507=VECTOR ( 'NONE', #1579, 1000.000000000000000 ) ;
#14508=ADVANCED_FACE ( 'NONE', ( #21576 ), #1629, .T. ) ;
#14511=CARTESIAN_POINT ( 'NONE',  ( 91.18044947428789726, 112.7436279071541776, 90.00000000000000000 ) ) ;
#14514=CARTESIAN_POINT ( 'NONE',  ( 160.0000000000000000, 1.959434878635765210E-14, 100.0000000000000000 ) ) ;
#14517=CIRCLE ( 'NONE', #12221, 7.500000000000000888 ) ;
#14523=CARTESIAN_POINT ( 'NONE',  ( -137.9031948627974486, 44.80746418436699940, -90.00000000000000000 ) ) ;
#14524=EDGE_CURVE ( 'NONE', #19753, #18149, #14020, .T. ) ;
#14545=ORIENTED_EDGE ( 'NONE', *, *, #15493, .T. ) ;
#14557=DIRECTION ( 'NONE',  ( 1.000000000000000000, 0.000000000000000000, 0.000000000000000000 ) ) ;
#14568=ORIENTED_EDGE ( 'NONE', *, *, #5050, .T. ) ;
#14574=( NAMED_UNIT ( * ) PLANE_ANGLE_UNIT ( ) SI_UNIT ( $, .RADIAN. ) );
#14592=EDGE_CURVE ( 'NONE', #22764, #17672, #1910, .T. ) ;
#14605=CARTESIAN_POINT ( 'NONE',  ( -85.22886158240879695, 117.3074641843673049, -90.00000000000000000 ) ) ;
#14606=ORIENTED_EDGE ( 'NONE', *, *, #12558, .T. ) ;
#14624=EDGE_CURVE ( 'NONE', #7615, #21317, #764, .T. ) ;
#14627=( GEOMETRIC_REPRESENTATION_CONTEXT ( 3 ) GLOBAL_UNCERTAINTY_ASSIGNED_CONTEXT ( ( #22948 ) ) GLOBAL_UNIT_ASSIGNED_CONTEXT ( ( #10972, #14574, #20220 ) ) REPRESENTATION_CONTEXT ( 'NONE', 'WORKASPACE' ) );
#14630=CIRCLE ( 'NONE', #20783, 7.500000000000005329 ) ;
#14638=EDGE_CURVE ( 'NONE', #1322, #16743, #12218, .T. ) ;
#14675=STYLED_ITEM ( 'NONE', ( #285 ), #11926 ) ;
#14680=CARTESIAN_POINT ( 'NONE',  ( 44.80746418436557832, 137.9031948627978750, -90.00000000000000000 ) ) ;
#14684=EDGE_CURVE ( 'NONE', #23301, #17463, #21108, .T. ) ;
#14688=CARTESIAN_POINT ( 'NONE',  ( -51.87806360044718446, -135.4018704341559953, -90.00000000000000000 ) ) ;
#14697=LINE ( 'NONE', #7066, #8418 ) ;
#14716=DIRECTION ( 'NONE',  ( 1.000000000000000000, 0.000000000000000000, 0.000000000000000000 ) ) ;
#14719=CARTESIAN_POINT ( 'NONE',  ( 0.000000000000000000, 0.000000000000000000, 100.0000000000000000 ) ) ;
#14720=VERTEX_POINT ( 'NONE', #7329 ) ;
#14734=EDGE_CURVE ( 'NONE', #22784, #9608, #15447, .T. ) ;
#14747=CARTESIAN_POINT ( 'NONE',  ( 35.00000000000000711, 0.000000000000000000, 100.0000000000000000 ) ) ;
#14765=VECTOR ( 'NONE', #7817, 1000.000000000000000 ) ;
#14767=EDGE_LOOP ( 'NONE', ( #3185, #8107, #6362, #12989, #15615, #13012 ) ) ;
#14775=ORIENTED_EDGE ( 'NONE', *, *, #15968, .F. ) ;
#14793=CARTESIAN_POINT ( 'NONE',  ( -137.5000000000000000, -5.062647941322544249E-13, 90.00000000000000000 ) ) ;
#14835=CARTESIAN_POINT ( 'NONE',  ( 37.61698748598423947, 140.0355749532214702, 90.00000000000000000 ) ) ;
#14843=ORIENTED_EDGE ( 'NONE', *, *, #8935, .F. ) ;
#14845=FACE_OUTER_BOUND ( 'NONE', #20828, .T. ) ;
#14875=AXIS2_PLACEMENT_3D ( 'NONE', #4488, #6415, #21272 ) ;
#14892=ORIENTED_EDGE ( 'NONE', *, *, #20230, .F. ) ;
#14894=DIRECTION ( 'NONE',  ( -1.000000000000000000, 0.000000000000000000, 0.000000000000000000 ) ) ;
#14909=LINE ( 'NONE', #2077, #369 ) ;
#14914=DIRECTION ( 'NONE',  ( 0.000000000000000000, 0.000000000000000000, 1.000000000000000000 ) ) ;
#14922=DIRECTION ( 'NONE',  ( -0.000000000000000000, -0.000000000000000000, 1.000000000000000000 ) ) ;
#14924=VECTOR ( 'NONE', #12612, 1000.000000000000000 ) ;
#14927=DIRECTION ( 'NONE',  ( -0.000000000000000000, -0.000000000000000000, 1.000000000000000000 ) ) ;
#14939=EDGE_CURVE ( 'NONE', #11303, #14252, #2483, .T. ) ;
#14960=CIRCLE ( 'NONE', #13826, 7.499999999999998224 ) ;
#14962=ORIENTED_EDGE ( 'NONE', *, *, #23189, .F. ) ;
#14965=CIRCLE ( 'NONE', #11512, 7.500000000000000888 ) ;
#14968=ORIENTED_EDGE ( 'NONE', *, *, #4517, .T. ) ;
#14983=AXIS2_PLACEMENT_3D ( 'NONE', #554, #11815, #19005 ) ;
#14987=CARTESIAN_POINT ( 'NONE',  ( 117.3074641843663386, 85.22886158241004750, 90.00000000000000000 ) ) ;
#14998=AXIS2_PLACEMENT_3D ( 'NONE', #16947, #15152, #17068 ) ;
#15006=AXIS2_PLACEMENT_3D ( 'NONE', #2957, #8196, #21225 ) ;
#15012=AXIS2_PLACEMENT_3D ( 'NONE', #14364, #20112, #12676 ) ;
#15017=AXIS2_PLACEMENT_3D ( 'NONE', #10325, #15994, #17669 ) ;
#15046=CARTESIAN_POINT ( 'NONE',  ( 121.5574576620388143, 79.04925354955381067, -90.00000000000000000 ) ) ;
#15055=VECTOR ( 'NONE', #16099, 1000.000000000000000 ) ;
#15069=DIRECTION ( 'NONE',  ( -0.000000000000000000, -0.000000000000000000, 1.000000000000000000 ) ) ;
#15074=EDGE_LOOP ( 'NONE', ( #23796, #1582, #12711, #18101 ) ) ;
#15090=ADVANCED_FACE ( 'NONE', ( #19261 ), #10228, .T. ) ;
#15142=ADVANCED_FACE ( 'NONE', ( #10483 ), #906, .T. ) ;
#15143=DIRECTION ( 'NONE',  ( 1.000000000000000000, 0.000000000000000000, 0.000000000000000000 ) ) ;
#15152=DIRECTION ( 'NONE',  ( 0.000000000000000000, -1.000000000000000000, 0.000000000000000000 ) ) ;
#15159=DIRECTION ( 'NONE',  ( 0.000000000000000000, 0.000000000000000000, 1.000000000000000000 ) ) ;
#15167=DIRECTION ( 'NONE',  ( 0.9510565162951534202, 0.3090169943749478398, 0.000000000000000000 ) ) ;
#15171=CARTESIAN_POINT ( 'NONE',  ( 121.5574576620388143, 79.04925354955381067, 90.00000000000000000 ) ) ;
#15181=DIRECTION ( 'NONE',  ( 0.000000000000000000, 0.000000000000000000, 1.000000000000000000 ) ) ;
#15184=ADVANCED_FACE ( 'NONE', ( #21676 ), #21560, .T. ) ;
#15185=DIRECTION ( 'NONE',  ( 0.000000000000000000, 0.000000000000000000, 1.000000000000000000 ) ) ;
#15189=DIRECTION ( 'NONE',  ( 0.000000000000000000, 0.000000000000000000, 1.000000000000000000 ) ) ;
#15191=ORIENTED_EDGE ( 'NONE', *, *, #21253, .T. ) ;
#15193=PLANE ( 'NONE',  #13947 ) ;
#15194=CARTESIAN_POINT ( 'NONE',  ( 0.000000000000000000, 0.000000000000000000, 90.00000000000000000 ) ) ;
#15222=ORIENTED_EDGE ( 'NONE', *, *, #21071, .T. ) ;
#15230=CARTESIAN_POINT ( 'NONE',  ( 0.000000000000000000, 0.000000000000000000, -90.00000000000000000 ) ) ;
#15235=EDGE_CURVE ( 'NONE', #11911, #5651, #399, .T. ) ;
#15241=ADVANCED_FACE ( 'NONE', ( #536 ), #649, .T. ) ;
#15248=EDGE_CURVE ( 'NONE', #4937, #4516, #6560, .T. ) ;
#15258=ORIENTED_EDGE ( 'NONE', *, *, #7243, .F. ) ;
#15263=VERTEX_POINT ( 'NONE', #15046 ) ;
#15287=AXIS2_PLACEMENT_3D ( 'NONE', #13480, #22836, #4258 ) ;
#15309=FACE_OUTER_BOUND ( 'NONE', #23743, .T. ) ;
#15359=FACE_OUTER_BOUND ( 'NONE', #22719, .T. ) ;
#15367=ORIENTED_EDGE ( 'NONE', *, *, #15248, .F. ) ;
#15374=EDGE_CURVE ( 'NONE', #9321, #15709, #17001, .T. ) ;
#15377=CARTESIAN_POINT ( 'NONE',  ( -37.61698748598617215, 140.0355749532209586, 90.00000000000000000 ) ) ;
#15378=AXIS2_PLACEMENT_3D ( 'NONE', #6251, #11602, #22786 ) ;
#15383=EDGE_CURVE ( 'NONE', #14205, #20274, #6565, .T. ) ;
#15407=CARTESIAN_POINT ( 'NONE',  ( 112.7436279071518612, 91.18044947429076785, -90.00000000000000000 ) ) ;
#15409=CARTESIAN_POINT ( 'NONE',  ( -140.0355749532208449, -37.61698748598668374, -90.00000000000000000 ) ) ;
#15411=AXIS2_PLACEMENT_3D ( 'NONE', #17093, #666, #19128 ) ;
#15415=ADVANCED_FACE ( 'NONE', ( #6679 ), #6209, .F. ) ;
#15447=CIRCLE ( 'NONE', #15821, 145.0000000000000284 ) ;
#15476=ORIENTED_EDGE ( 'NONE', *, *, #8980, .F. ) ;
#15477=DIRECTION ( 'NONE',  ( -0.8090169943749428993, -0.5877852522924793544, 0.000000000000000000 ) ) ;
#15493=EDGE_CURVE ( 'NONE', #10493, #13502, #2803, .T. ) ;
#15499=ORIENTED_EDGE ( 'NONE', *, *, #13067, .T. ) ;
#15508=EDGE_CURVE ( 'NONE', #21395, #1131, #18910, .T. ) ;
#15536=DIRECTION ( 'NONE',  ( -0.000000000000000000, -0.000000000000000000, -1.000000000000000000 ) ) ;
#15537=CARTESIAN_POINT ( 'NONE',  ( 7.499999999999997335, 34.18698582794336005, -100.0000000000000000 ) ) ;
#15543=DIRECTION ( 'NONE',  ( 1.000000000000000000, 0.000000000000000000, 0.000000000000000000 ) ) ;
#15544=CARTESIAN_POINT ( 'NONE',  ( 0.000000000000000000, 0.000000000000000000, -100.0000000000000000 ) ) ;
#15615=ORIENTED_EDGE ( 'NONE', *, *, #20073, .F. ) ;
#15618=ORIENTED_EDGE ( 'NONE', *, *, #19927, .F. ) ;
#15632=CARTESIAN_POINT ( 'NONE',  ( 7.499999999999999112, 41.99999999999998579, -100.0000000000000000 ) ) ;
#15636=EDGE_LOOP ( 'NONE', ( #2684, #17120, #9363, #12433 ) ) ;
#15656=DIRECTION ( 'NONE',  ( 0.000000000000000000, -0.000000000000000000, 1.000000000000000000 ) ) ;
#15664=DIRECTION ( 'NONE',  ( -0.000000000000000000, -0.000000000000000000, 1.000000000000000000 ) ) ;
#15666=AXIS2_PLACEMENT_3D ( 'NONE', #8035, #2351, #440 ) ;
#15667=ORIENTED_EDGE ( 'NONE', *, *, #2575, .T. ) ;
#15668=CARTESIAN_POINT ( 'NONE',  ( 7.499999999999999112, 41.99999999999998579, -100.0000000000000000 ) ) ;
#15686=DIRECTION ( 'NONE',  ( 0.000000000000000000, -0.000000000000000000, -1.000000000000000000 ) ) ;
#15699=DIRECTION ( 'NONE',  ( 0.000000000000000000, 0.000000000000000000, 1.000000000000000000 ) ) ;
#15703=ORIENTED_EDGE ( 'NONE', *, *, #20391, .T. ) ;
#15704=AXIS2_PLACEMENT_3D ( 'NONE', #3370, #14164, #3497 ) ;
#15708=ORIENTED_EDGE ( 'NONE', *, *, #2032, .T. ) ;
#15709=VERTEX_POINT ( 'NONE', #9810 ) ;
#15730=ORIENTED_EDGE ( 'NONE', *, *, #4782, .F. ) ;
#15737=DIRECTION ( 'NONE',  ( 0.000000000000000000, 0.000000000000000000, 1.000000000000000000 ) ) ;
#15751=AXIS2_PLACEMENT_3D ( 'NONE', #15896, #23469, #19366 ) ;
#15763=CARTESIAN_POINT ( 'NONE',  ( 85.22886158240706322, 117.3074641843685129, -90.00000000000000000 ) ) ;
#15770=CIRCLE ( 'NONE', #333, 7.500000000000003553 ) ;
#15788=AXIS2_PLACEMENT_3D ( 'NONE', #23229, #4884, #12292 ) ;
#15821=AXIS2_PLACEMENT_3D ( 'NONE', #3685, #16637, #14716 ) ;
#15825=FACE_OUTER_BOUND ( 'NONE', #402, .T. ) ;
#15828=ORIENTED_EDGE ( 'NONE', *, *, #11719, .F. ) ;
#15842=AXIS2_PLACEMENT_3D ( 'NONE', #3543, #5027, #14557 ) ;
#15852=VECTOR ( 'NONE', #17795, 1000.000000000000000 ) ;
#15855=ADVANCED_FACE ( 'NONE', ( #12347 ), #16642, .F. ) ;
#15856=VERTEX_POINT ( 'NONE', #14835 ) ;
#15877=DIRECTION ( 'NONE',  ( 1.000000000000000000, 0.000000000000000000, 0.000000000000000000 ) ) ;
#15887=DIRECTION ( 'NONE',  ( -0.3090169943749517811, 0.9510565162951520879, 0.000000000000000000 ) ) ;
#15890=DIRECTION ( 'NONE',  ( 0.000000000000000000, -0.000000000000000000, 1.000000000000000000 ) ) ;
#15896=CARTESIAN_POINT ( 'NONE',  ( 44.80746418436846312, -137.9031948627969655, -90.00000000000000000 ) ) ;
#15913=ORIENTED_EDGE ( 'NONE', *, *, #13058, .F. ) ;
#15927=EDGE_LOOP ( 'NONE', ( #12083, #17884, #121, #519 ) ) ;
#15942=EDGE_CURVE ( 'NONE', #10771, #17172, #13853, .T. ) ;
#15955=CARTESIAN_POINT ( 'NONE',  ( 0.000000000000000000, 0.000000000000000000, 90.00000000000000000 ) ) ;
#15964=ORIENTED_EDGE ( 'NONE', *, *, #23189, .T. ) ;
#15968=EDGE_CURVE ( 'NONE', #14720, #2646, #4558, .T. ) ;
#15971=DIRECTION ( 'NONE',  ( 1.000000000000000000, 0.000000000000000000, 0.000000000000000000 ) ) ;
#15977=CARTESIAN_POINT ( 'NONE',  ( 0.000000000000000000, 0.000000000000000000, 90.00000000000000000 ) ) ;
#15994=DIRECTION ( 'NONE',  ( 0.000000000000000000, 0.000000000000000000, 1.000000000000000000 ) ) ;
#16018=EDGE_LOOP ( 'NONE', ( #6155, #21813, #22451, #11983 ) ) ;
#16032=LINE ( 'NONE', #23381, #22902 ) ;
#16040=LINE ( 'NONE', #4563, #8227 ) ;
#16045=LINE ( 'NONE', #23522, #9549 ) ;
#16046=CARTESIAN_POINT ( 'NONE',  ( -144.8060344827586619, 7.497491405671214082, -2.775557561562891351E-14 ) ) ;
#16060=LINE ( 'NONE', #23758, #23268 ) ;
#16075=ADVANCED_FACE ( 'NONE', ( #22416 ), #7813, .F. ) ;
#16077=EDGE_CURVE ( 'NONE', #14252, #3378, #19587, .T. ) ;
#16078=LINE ( 'NONE', #2667, #20237 ) ;
#16095=EDGE_CURVE ( 'NONE', #17693, #1131, #11924, .T. ) ;
#16099=DIRECTION ( 'NONE',  ( -0.000000000000000000, -0.000000000000000000, 1.000000000000000000 ) ) ;
#16121=DIRECTION ( 'NONE',  ( 0.000000000000000000, 0.000000000000000000, 1.000000000000000000 ) ) ;
#16126=DIRECTION ( 'NONE',  ( 0.000000000000000000, 0.000000000000000000, 1.000000000000000000 ) ) ;
#16150=CARTESIAN_POINT ( 'NONE',  ( -144.8060344827586619, 7.497491405671214082, 90.00000000000000000 ) ) ;
#16153=CARTESIAN_POINT ( 'NONE',  ( 0.000000000000000000, 0.000000000000000000, -90.00000000000000000 ) ) ;
#16160=DIRECTION ( 'NONE',  ( 0.000000000000000000, 0.000000000000000000, 1.000000000000000000 ) ) ;
#16165=CARTESIAN_POINT ( 'NONE',  ( -7.497491405671719455, -144.8060344827586334, -2.775557561562891351E-14 ) ) ;
#16170=AXIS2_PLACEMENT_3D ( 'NONE', #3407, #23585, #21768 ) ;
#16188=AXIS2_PLACEMENT_3D ( 'NONE', #16351, #7160, #21886 ) ;
#16192=AXIS2_PLACEMENT_3D ( 'NONE', #12539, #23120, #19967 ) ;
#16195=LINE ( 'NONE', #12239, #18594 ) ;
#16208=VECTOR ( 'NONE', #14187, 1000.000000000000000 ) ;
#16213=CYLINDRICAL_SURFACE ( 'NONE', #2874, 7.500000000000007105 ) ;
#16228=AXIS2_PLACEMENT_3D ( 'NONE', #17839, #4918, #10504 ) ;
#16232=CYLINDRICAL_SURFACE ( 'NONE', #16598, 7.500000000000007105 ) ;
#16234=ORIENTED_EDGE ( 'NONE', *, *, #18170, .T. ) ;
#16238=ORIENTED_EDGE ( 'NONE', *, *, #2636, .T. ) ;
#16255=DIRECTION ( 'NONE',  ( 0.000000000000000000, 0.000000000000000000, 1.000000000000000000 ) ) ;
#16258=CARTESIAN_POINT ( 'NONE',  ( 79.04925354955338435, -121.5574576620390843, -90.00000000000000000 ) ) ;
#16267=ORIENTED_EDGE ( 'NONE', *, *, #6601, .F. ) ;
#16273=CARTESIAN_POINT ( 'NONE',  ( 137.9031948627967950, 44.80746418436894629, -90.00000000000000000 ) ) ;
#16282=DIRECTION ( 'NONE',  ( -0.8090169943749507819, 0.5877852522924686962, 0.000000000000000000 ) ) ;
#16301=DIRECTION ( 'NONE',  ( 1.000000000000000000, 0.000000000000000000, 0.000000000000000000 ) ) ;
#16306=AXIS2_PLACEMENT_3D ( 'NONE', #11466, #13770, #21089 ) ;
#16320=CARTESIAN_POINT ( 'NONE',  ( -117.3074641843675749, 85.22886158240835641, -90.00000000000000000 ) ) ;
#16338=ORIENTED_EDGE ( 'NONE', *, *, #6633, .F. ) ;
#16341=CIRCLE ( 'NONE', #5148, 7.500000000000000888 ) ;
#16343=EDGE_LOOP ( 'NONE', ( #6649, #599, #20946, #14892 ) ) ;
#16351=CARTESIAN_POINT ( 'NONE',  ( 137.9031948627967950, 44.80746418436894629, 90.00000000000000000 ) ) ;
#16356=( LENGTH_UNIT ( ) NAMED_UNIT ( * ) SI_UNIT ( .MILLI., .METRE. ) );
#16360=CARTESIAN_POINT ( 'NONE',  ( 7.497491405671719455, -144.8060344827586334, -90.00000000000000000 ) ) ;
#16381=CARTESIAN_POINT ( 'NONE',  ( -117.3074641843669781, -85.22886158240918064, -90.00000000000000000 ) ) ;
#16387=CIRCLE ( 'NONE', #18618, 35.00000000000000711 ) ;
#16391=ORIENTED_EDGE ( 'NONE', *, *, #17170, .F. ) ;
#16394=DIRECTION ( 'NONE',  ( 1.000000000000000000, 0.000000000000000000, 0.000000000000000000 ) ) ;
#16410=CARTESIAN_POINT ( 'NONE',  ( 7.497491405671719455, -144.8060344827586334, -2.775557561562891351E-14 ) ) ;
#16429=ADVANCED_FACE ( 'NONE', ( #9599 ), #6080, .F. ) ;
#16438=CARTESIAN_POINT ( 'NONE',  ( 0.000000000000000000, 0.000000000000000000, 90.00000000000000000 ) ) ;
#16457=CIRCLE ( 'NONE', #23773, 7.500000000000000000 ) ;
#16466=CARTESIAN_POINT ( 'NONE',  ( 144.8060344827585482, 7.497491405673235576, -2.775557561562891351E-14 ) ) ;
#16477=CIRCLE ( 'NONE', #21863, 145.0000000000000284 ) ;
#16478=EDGE_CURVE ( 'NONE', #9321, #11736, #2912, .T. ) ;
#16480=DIRECTION ( 'NONE',  ( 0.9510565162951534202, 0.3090169943749478398, 0.000000000000000000 ) ) ;
#16495=AXIS2_PLACEMENT_3D ( 'NONE', #13598, #4365, #14894 ) ;
#16496=EDGE_CURVE ( 'NONE', #13908, #23165, #9482, .T. ) ;
#16497=DIRECTION ( 'NONE',  ( 1.000000000000000000, 0.000000000000000000, 0.000000000000000000 ) ) ;
#16501=VERTEX_POINT ( 'NONE', #4389 ) ;
#16539=AXIS2_PLACEMENT_3D ( 'NONE', #21392, #23568, #6786 ) ;
#16542=CIRCLE ( 'NONE', #15006, 7.500000000000000000 ) ;
#16546=LINE ( 'NONE', #14514, #14507 ) ;
#16552=CIRCLE ( 'NONE', #6145, 145.0000000000000284 ) ;
#16553=CARTESIAN_POINT ( 'NONE',  ( -51.87806360044816500, 135.4018704341555974, 90.00000000000000000 ) ) ;
#16565=ORIENTED_EDGE ( 'NONE', *, *, #3241, .F. ) ;
#16567=CYLINDRICAL_SURFACE ( 'NONE', #4537, 160.0000000000000000 ) ;
#16571=ORIENTED_EDGE ( 'NONE', *, *, #9791, .T. ) ;
#16572=ORIENTED_EDGE ( 'NONE', *, *, #20620, .F. ) ;
#16598=AXIS2_PLACEMENT_3D ( 'NONE', #1595, #10808, #19943 ) ;
#16600=CIRCLE ( 'NONE', #18512, 145.0000000000000284 ) ;
#16617=AXIS2_PLACEMENT_3D ( 'NONE', #10017, #10252, #8200 ) ;
#16619=CARTESIAN_POINT ( 'NONE',  ( -44.80746418436748968, 137.9031948627972781, 90.00000000000000000 ) ) ;
#16634=ORIENTED_EDGE ( 'NONE', *, *, #18145, .T. ) ;
#16637=DIRECTION ( 'NONE',  ( 0.000000000000000000, 0.000000000000000000, 1.000000000000000000 ) ) ;
#16642=CYLINDRICAL_SURFACE ( 'NONE', #19179, 7.500000000000007105 ) ;
#16651=LINE ( 'NONE', #16410, #1148 ) ;
#16665=CARTESIAN_POINT ( 'NONE',  ( 0.000000000000000000, 0.000000000000000000, 90.00000000000000000 ) ) ;
#16715=SURFACE_SIDE_STYLE ('',( #9115 ) ) ;
#16731=VECTOR ( 'NONE', #6035, 1000.000000000000000 ) ;
#16743=VERTEX_POINT ( 'NONE', #8739 ) ;
#16768=VECTOR ( 'NONE', #13957, 1000.000000000000000 ) ;
#16771=ORIENTED_EDGE ( 'NONE', *, *, #18856, .T. ) ;
#16773=PRODUCT_DEFINITION_CONTEXT ( 'detailed design', #12972, 'design' ) ;
#16785=ORIENTED_EDGE ( 'NONE', *, *, #991, .F. ) ;
#16786=CARTESIAN_POINT ( 'NONE',  ( -7.499999999999999112, 41.99999999999998579, 100.0000000000000000 ) ) ;
#16811=CIRCLE ( 'NONE', #17568, 7.500000000000000000 ) ;
#16812=CARTESIAN_POINT ( 'NONE',  ( -135.4018704341557964, 51.87806360044768894, -90.00000000000000000 ) ) ;
#16823=ORIENTED_EDGE ( 'NONE', *, *, #8783, .F. ) ;
#16826=FILL_AREA_STYLE ('',( #18272 ) ) ;
#16863=DIRECTION ( 'NONE',  ( 0.000000000000000000, 0.000000000000000000, 1.000000000000000000 ) ) ;
#16873=LINE ( 'NONE', #7820, #12203 ) ;
#16893=CIRCLE ( 'NONE', #23053, 7.500000000000000000 ) ;
#16900=EDGE_LOOP ( 'NONE', ( #8455, #4119, #22819, #17583 ) ) ;
#16902=ORIENTED_EDGE ( 'NONE', *, *, #21837, .F. ) ;
#16913=CARTESIAN_POINT ( 'NONE',  ( -77.72886158240795851, -117.3074641843678876, -90.00000000000000000 ) ) ;
#16919=CARTESIAN_POINT ( 'NONE',  ( 0.000000000000000000, 0.000000000000000000, -90.00000000000000000 ) ) ;
#16940=LINE ( 'NONE', #13474, #10419 ) ;
#16943=ORIENTED_EDGE ( 'NONE', *, *, #21410, .T. ) ;
#16947=CARTESIAN_POINT ( 'NONE',  ( -7.499999999999999112, 41.99999999999998579, -100.0000000000000000 ) ) ;
#16954=AXIS2_PLACEMENT_3D ( 'NONE', #5128, #16255, #6591 ) ;
#16960=FACE_OUTER_BOUND ( 'NONE', #15074, .T. ) ;
#16970=DIRECTION ( 'NONE',  ( 0.000000000000000000, 0.000000000000000000, 1.000000000000000000 ) ) ;
#16980=ADVANCED_FACE ( 'NONE', ( #1577 ), #18341, .F. ) ;
#16983=DIRECTION ( 'NONE',  ( 0.000000000000000000, 0.000000000000000000, -1.000000000000000000 ) ) ;
#16989=LINE ( 'NONE', #7675, #9614 ) ;
#16990=EDGE_CURVE ( 'NONE', #13461, #19833, #20152, .T. ) ;
#17001=CIRCLE ( 'NONE', #3489, 7.500000000000000888 ) ;
#17027=FACE_OUTER_BOUND ( 'NONE', #10153, .T. ) ;
#17028=CARTESIAN_POINT ( 'NONE',  ( -112.7436279071525433, -91.18044947428992941, -90.00000000000000000 ) ) ;
#17056=VERTEX_POINT ( 'NONE', #14511 ) ;
#17058=DIRECTION ( 'NONE',  ( 0.8090169943749468962, 0.5877852522924740253, 0.000000000000000000 ) ) ;
#17068=DIRECTION ( 'NONE',  ( 0.000000000000000000, -0.000000000000000000, -1.000000000000000000 ) ) ;
#17087=EDGE_LOOP ( 'NONE', ( #4248, #20204, #20663, #7176 ) ) ;
#17093=CARTESIAN_POINT ( 'NONE',  ( 0.000000000000000000, 0.000000000000000000, -90.00000000000000000 ) ) ;
#17096=CARTESIAN_POINT ( 'NONE',  ( 0.000000000000000000, 0.000000000000000000, -100.0000000000000000 ) ) ;
#17120=ORIENTED_EDGE ( 'NONE', *, *, #10223, .T. ) ;
#17133=AXIS2_PLACEMENT_3D ( 'NONE', #16153, #3207, #8791 ) ;
#17143=ORIENTED_EDGE ( 'NONE', *, *, #10223, .F. ) ;
#17170=EDGE_CURVE ( 'NONE', #11696, #11121, #7988, .T. ) ;
#17172=VERTEX_POINT ( 'NONE', #14747 ) ;
#17174=EDGE_CURVE ( 'NONE', #16501, #17172, #20267, .T. ) ;
#17216=ORIENTED_EDGE ( 'NONE', *, *, #20939, .F. ) ;
#17233=DIRECTION ( 'NONE',  ( 0.3090169943749441761, 0.9510565162951546414, 0.000000000000000000 ) ) ;
#17240=EDGE_CURVE ( 'NONE', #20139, #13908, #11097, .T. ) ;
#17242=ORIENTED_EDGE ( 'NONE', *, *, #6169, .F. ) ;
#17258=DIRECTION ( 'NONE',  ( -0.000000000000000000, -0.000000000000000000, 1.000000000000000000 ) ) ;
#17261=ORIENTED_EDGE ( 'NONE', *, *, #4759, .T. ) ;
#17268=CARTESIAN_POINT ( 'NONE',  ( 144.8060344827587187, -7.497491405670202447, 90.00000000000000000 ) ) ;
#17281=ADVANCED_FACE ( 'NONE', ( #6386 ), #13793, .F. ) ;
#17284=AXIS2_PLACEMENT_3D ( 'NONE', #9703, #5828, #17058 ) ;
#17292=ORIENTED_EDGE ( 'NONE', *, *, #20157, .F. ) ;
#17296=DIRECTION ( 'NONE',  ( 0.9510565162951534202, 0.3090169943749478398, 0.000000000000000000 ) ) ;
#17310=LINE ( 'NONE', #6424, #12352 ) ;
#17321=AXIS2_PLACEMENT_3D ( 'NONE', #10203, #4875, #2710 ) ;
#17337=FACE_OUTER_BOUND ( 'NONE', #10400, .T. ) ;
#17340=CIRCLE ( 'NONE', #2283, 145.0000000000000284 ) ;
#17342=( GEOMETRIC_REPRESENTATION_CONTEXT ( 3 ) GLOBAL_UNCERTAINTY_ASSIGNED_CONTEXT ( ( #21033 ) ) GLOBAL_UNIT_ASSIGNED_CONTEXT ( ( #2083, #18169, #22380 ) ) REPRESENTATION_CONTEXT ( 'NONE', 'WORKASPACE' ) );
#17350=DIRECTION ( 'NONE',  ( 0.000000000000000000, 0.000000000000000000, 1.000000000000000000 ) ) ;
#17357=ORIENTED_EDGE ( 'NONE', *, *, #5050, .F. ) ;
#17366=VECTOR ( 'NONE', #7864, 1000.000000000000000 ) ;
#17389=CARTESIAN_POINT ( 'NONE',  ( 0.000000000000000000, 0.000000000000000000, -90.00000000000000000 ) ) ;
#17391=ORIENTED_EDGE ( 'NONE', *, *, #22603, .F. ) ;
#17392=DIRECTION ( 'NONE',  ( -0.3090169943749517811, 0.9510565162951520879, 0.000000000000000000 ) ) ;
#17393=CARTESIAN_POINT ( 'NONE',  ( -44.80746418436748968, 137.9031948627972781, -90.00000000000000000 ) ) ;
#17394=CARTESIAN_POINT ( 'NONE',  ( -85.22886158240795851, -117.3074641843678876, 90.00000000000000000 ) ) ;
#17395=EDGE_LOOP ( 'NONE', ( #19263, #15191, #22557, #5827 ) ) ;
#17416=DIRECTION ( 'NONE',  ( 0.000000000000000000, 0.000000000000000000, 1.000000000000000000 ) ) ;
#17417=EDGE_LOOP ( 'NONE', ( #2459, #14132 ) ) ;
#17422=UNCERTAINTY_MEASURE_WITH_UNIT (LENGTH_MEASURE( 1.000000000000000082E-05 ), #16356, 'distance_accuracy_value', 'NONE');
#17423=FACE_OUTER_BOUND ( 'NONE', #12836, .T. ) ;
#17425=CARTESIAN_POINT ( 'NONE',  ( 140.0355749532205607, 37.61698748598765718, 90.00000000000000000 ) ) ;
#17444=EDGE_CURVE ( 'NONE', #4114, #20274, #6046, .T. ) ;
#17463=VERTEX_POINT ( 'NONE', #21823 ) ;
#17500=ORIENTED_EDGE ( 'NONE', *, *, #22472, .F. ) ;
#17517=LINE ( 'NONE', #2676, #595 ) ;
#17527=CYLINDRICAL_SURFACE ( 'NONE', #10365, 145.0000000000000284 ) ;
#17531=CARTESIAN_POINT ( 'NONE',  ( 0.000000000000000000, 0.000000000000000000, 90.00000000000000000 ) ) ;
#17541=CARTESIAN_POINT ( 'NONE',  ( -35.00000000000000711, 4.286263797015737285E-15, 100.0000000000000000 ) ) ;
#17568=AXIS2_PLACEMENT_3D ( 'NONE', #9911, #20626, #15477 ) ;
#17571=EDGE_CURVE ( 'NONE', #13321, #8675, #14965, .T. ) ;
#17575=CARTESIAN_POINT ( 'NONE',  ( 117.3074641843663386, 85.22886158241004750, -90.00000000000000000 ) ) ;
#17583=ORIENTED_EDGE ( 'NONE', *, *, #4759, .F. ) ;
#17608=ORIENTED_EDGE ( 'NONE', *, *, #13798, .F. ) ;
#17613=DIRECTION ( 'NONE',  ( 0.000000000000000000, 0.000000000000000000, 1.000000000000000000 ) ) ;
#17614=DIRECTION ( 'NONE',  ( 0.000000000000000000, 0.000000000000000000, -1.000000000000000000 ) ) ;
#17622=VERTEX_POINT ( 'NONE', #13621 ) ;
#17651=ORIENTED_EDGE ( 'NONE', *, *, #19929, .F. ) ;
#17661=AXIS2_PLACEMENT_3D ( 'NONE', #16438, #4977, #23789 ) ;
#17669=DIRECTION ( 'NONE',  ( 1.110223024625156383E-14, -1.000000000000000000, 0.000000000000000000 ) ) ;
#17672=VERTEX_POINT ( 'NONE', #10994 ) ;
#17679=DIRECTION ( 'NONE',  ( 1.000000000000000000, 0.000000000000000000, 0.000000000000000000 ) ) ;
#17692=VERTEX_POINT ( 'NONE', #8507 ) ;
#17693=VERTEX_POINT ( 'NONE', #19714 ) ;
#17709=DIRECTION ( 'NONE',  ( 1.000000000000000000, 0.000000000000000000, 0.000000000000000000 ) ) ;
#17723=EDGE_LOOP ( 'NONE', ( #12200, #63, #18400, #3429 ) ) ;
#17727=DIRECTION ( 'NONE',  ( 1.000000000000000000, 0.000000000000000000, 0.000000000000000000 ) ) ;
#17735=DIRECTION ( 'NONE',  ( 1.000000000000000000, 0.000000000000000000, 0.000000000000000000 ) ) ;
#17746=VERTEX_POINT ( 'NONE', #19350 ) ;
#17750=CARTESIAN_POINT ( 'NONE',  ( -37.30746418436748968, 137.9031948627972781, -90.00000000000000000 ) ) ;
#17761=AXIS2_PLACEMENT_3D ( 'NONE', #1267, #1016, #8398 ) ;
#17771=VECTOR ( 'NONE', #6433, 1000.000000000000000 ) ;
#17772=EDGE_LOOP ( 'NONE', ( #16238, #13837, #4404, #14843 ) ) ;
#17785=CARTESIAN_POINT ( 'NONE',  ( 121.5574576620405480, -79.04925354955113903, -90.00000000000000000 ) ) ;
#17791=ORIENTED_EDGE ( 'NONE', *, *, #16496, .F. ) ;
#17795=DIRECTION ( 'NONE',  ( -0.000000000000000000, -0.000000000000000000, 1.000000000000000000 ) ) ;
#17813=CARTESIAN_POINT ( 'NONE',  ( -7.497491405671719455, 144.8060344827586334, -90.00000000000000000 ) ) ;
#17828=ORIENTED_EDGE ( 'NONE', *, *, #13547, .T. ) ;
#17834=EDGE_CURVE ( 'NONE', #4754, #9308, #4535, .T. ) ;
#17839=CARTESIAN_POINT ( 'NONE',  ( -137.9031948627974486, 44.80746418436699940, 90.00000000000000000 ) ) ;
#17853=ORIENTED_EDGE ( 'NONE', *, *, #16095, .F. ) ;
#17860=DIRECTION ( 'NONE',  ( 0.000000000000000000, 0.000000000000000000, 1.000000000000000000 ) ) ;
#17869=DIRECTION ( 'NONE',  ( 0.000000000000000000, 0.000000000000000000, 1.000000000000000000 ) ) ;
#17872=ORIENTED_EDGE ( 'NONE', *, *, #11142, .T. ) ;
#17884=ORIENTED_EDGE ( 'NONE', *, *, #8783, .T. ) ;
#17887=CARTESIAN_POINT ( 'NONE',  ( -85.22886158240879695, 117.3074641843673049, -90.00000000000000000 ) ) ;
#17894=EDGE_LOOP ( 'NONE', ( #15828, #19127, #23466, #20714 ) ) ;
#17907=CARTESIAN_POINT ( 'NONE',  ( 44.80746418436557832, 137.9031948627978750, -90.00000000000000000 ) ) ;
#17909=ORIENTED_EDGE ( 'NONE', *, *, #8034, .T. ) ;
#17926=FACE_OUTER_BOUND ( 'NONE', #17772, .T. ) ;
#17930=CARTESIAN_POINT ( 'NONE',  ( 0.000000000000000000, 0.000000000000000000, -90.00000000000000000 ) ) ;
#17944=DIRECTION ( 'NONE',  ( 0.000000000000000000, 0.000000000000000000, 1.000000000000000000 ) ) ;
#17955=FACE_OUTER_BOUND ( 'NONE', #3828, .T. ) ;
#17972=ORIENTED_EDGE ( 'NONE', *, *, #23208, .T. ) ;
#17975=CIRCLE ( 'NONE', #7550, 35.00000000000000711 ) ;
#18018=DIRECTION ( 'NONE',  ( 0.000000000000000000, 0.000000000000000000, 1.000000000000000000 ) ) ;
#18029=EDGE_CURVE ( 'NONE', #6740, #21770, #3755, .T. ) ;
#18032=ORIENTED_EDGE ( 'NONE', *, *, #13607, .F. ) ;
#18036=DIRECTION ( 'NONE',  ( 1.000000000000000000, 0.000000000000000000, 0.000000000000000000 ) ) ;
#18041=ADVANCED_FACE ( 'NONE', ( #2314 ), #6188, .T. ) ;
#18062=DIRECTION ( 'NONE',  ( 0.000000000000000000, 0.000000000000000000, 1.000000000000000000 ) ) ;
#18071=VECTOR ( 'NONE', #4126, 1000.000000000000000 ) ;
#18074=AXIS2_PLACEMENT_3D ( 'NONE', #13962, #15737, #2441 ) ;
#18086=DIRECTION ( 'NONE',  ( 0.000000000000000000, 0.000000000000000000, 1.000000000000000000 ) ) ;
#18101=ORIENTED_EDGE ( 'NONE', *, *, #14119, .F. ) ;
#18115=AXIS2_PLACEMENT_3D ( 'NONE', #22869, #9983, #8173 ) ;
#18138=EDGE_CURVE ( 'NONE', #4268, #17746, #8318, .T. ) ;
#18145=EDGE_CURVE ( 'NONE', #7169, #3375, #213, .T. ) ;
#18149=VERTEX_POINT ( 'NONE', #8347 ) ;
#18161=VERTEX_POINT ( 'NONE', #14053 ) ;
#18169=( NAMED_UNIT ( * ) PLANE_ANGLE_UNIT ( ) SI_UNIT ( $, .RADIAN. ) );
#18170=EDGE_CURVE ( 'NONE', #11764, #4268, #17517, .T. ) ;
#18176=EDGE_CURVE ( 'NONE', #880, #20274, #7919, .T. ) ;
#18184=VERTEX_POINT ( 'NONE', #856 ) ;
#18218=ORIENTED_EDGE ( 'NONE', *, *, #15508, .F. ) ;
#18252=ADVANCED_FACE ( 'NONE', ( #18801 ), #20615, .T. ) ;
#18272=FILL_AREA_STYLE_COLOUR ( '', #7717 ) ;
#18295=DIRECTION ( 'NONE',  ( -0.5877852522924773560, 0.8090169943749444537, 0.000000000000000000 ) ) ;
#18305=VERTEX_POINT ( 'NONE', #9779 ) ;
#18315=AXIS2_PLACEMENT_3D ( 'NONE', #8072, #466, #11469 ) ;
#18320=ORIENTED_EDGE ( 'NONE', *, *, #3849, .F. ) ;
#18323=ADVANCED_FACE ( 'NONE', ( #5797 ), #13676, .F. ) ;
#18334=ORIENTED_EDGE ( 'NONE', *, *, #18454, .F. ) ;
#18341=CYLINDRICAL_SURFACE ( 'NONE', #15704, 7.500000000000007105 ) ;
#18342=VERTEX_POINT ( 'NONE', #17028 ) ;
#18347=DIRECTION ( 'NONE',  ( -0.000000000000000000, -0.000000000000000000, 1.000000000000000000 ) ) ;
#18355=ADVANCED_FACE ( 'NONE', ( #13411 ), #2129, .F. ) ;
#18396=DIRECTION ( 'NONE',  ( -0.000000000000000000, -0.000000000000000000, 1.000000000000000000 ) ) ;
#18400=ORIENTED_EDGE ( 'NONE', *, *, #11514, .F. ) ;
#18407=EDGE_CURVE ( 'NONE', #5651, #5818, #16873, .T. ) ;
#18416=EDGE_LOOP ( 'NONE', ( #6809, #13875, #19720, #2579 ) ) ;
#18454=EDGE_CURVE ( 'NONE', #19875, #3015, #5228, .T. ) ;
#18483=ORIENTED_EDGE ( 'NONE', *, *, #9820, .T. ) ;
#18485=CARTESIAN_POINT ( 'NONE',  ( -44.80746418436648071, -137.9031948627975908, -90.00000000000000000 ) ) ;
#18488=ORIENTED_EDGE ( 'NONE', *, *, #9417, .F. ) ;
#18500=ADVANCED_FACE ( 'NONE', ( #6723 ), #21449, .T. ) ;
#18512=AXIS2_PLACEMENT_3D ( 'NONE', #11008, #12489, #20255 ) ;
#18531=ORIENTED_EDGE ( 'NONE', *, *, #15374, .T. ) ;
#18541=DIRECTION ( 'NONE',  ( 0.000000000000000000, 0.000000000000000000, 1.000000000000000000 ) ) ;
#18575=FACE_OUTER_BOUND ( 'NONE', #7273, .T. ) ;
#18590=CARTESIAN_POINT ( 'NONE',  ( -130.4031948627974486, 44.80746418436699940, 90.00000000000000000 ) ) ;
#18594=VECTOR ( 'NONE', #23049, 1000.000000000000000 ) ;
#18600=VERTEX_POINT ( 'NONE', #19278 ) ;
#18605=CARTESIAN_POINT ( 'NONE',  ( -145.0000000000000284, -5.062647941322544249E-13, -90.00000000000000000 ) ) ;
#18612=DIRECTION ( 'NONE',  ( 0.000000000000000000, -0.000000000000000000, 1.000000000000000000 ) ) ;
#18618=AXIS2_PLACEMENT_3D ( 'NONE', #13263, #20570, #9607 ) ;
#18622=DIRECTION ( 'NONE',  ( 1.000000000000000000, 0.000000000000000000, 0.000000000000000000 ) ) ;
#18637=DIRECTION ( 'NONE',  ( 0.000000000000000000, 0.000000000000000000, -1.000000000000000000 ) ) ;
#18642=CARTESIAN_POINT ( 'NONE',  ( 0.000000000000000000, 0.000000000000000000, -90.00000000000000000 ) ) ;
#18652=FACE_BOUND ( 'NONE', #14767, .T. ) ;
#18657=ORIENTED_EDGE ( 'NONE', *, *, #6215, .F. ) ;
#18672=VECTOR ( 'NONE', #8164, 1000.000000000000000 ) ;
#18683=ORIENTED_EDGE ( 'NONE', *, *, #13767, .T. ) ;
#18689=AXIS2_PLACEMENT_3D ( 'NONE', #19535, #17860, #19412 ) ;
#18694=ORIENTED_EDGE ( 'NONE', *, *, #3737, .T. ) ;
#18706=EDGE_CURVE ( 'NONE', #20079, #16743, #11046, .T. ) ;
#18722=DIRECTION ( 'NONE',  ( -0.000000000000000000, -0.000000000000000000, 1.000000000000000000 ) ) ;
#18723=DIRECTION ( 'NONE',  ( 1.000000000000000000, 0.000000000000000000, 0.000000000000000000 ) ) ;
#18734=AXIS2_PLACEMENT_3D ( 'NONE', #7531, #20930, #7780 ) ;
#18753=CARTESIAN_POINT ( 'NONE',  ( -7.497491405671719455, 144.8060344827586334, 90.00000000000000000 ) ) ;
#18763=DIRECTION ( 'NONE',  ( -0.3090169943749517811, 0.9510565162951520879, 0.000000000000000000 ) ) ;
#18775=CARTESIAN_POINT ( 'NONE',  ( 0.000000000000000000, 0.000000000000000000, 90.00000000000000000 ) ) ;
#18778=ORIENTED_EDGE ( 'NONE', *, *, #17240, .F. ) ;
#18801=FACE_OUTER_BOUND ( 'NONE', #8178, .T. ) ;
#18828=CARTESIAN_POINT ( 'NONE',  ( -77.72886158240878274, 117.3074641843673049, 90.00000000000000000 ) ) ;
#18842=AXIS2_PLACEMENT_3D ( 'NONE', #9626, #18541, #5399 ) ;
#18856=EDGE_CURVE ( 'NONE', #9872, #1295, #14517, .T. ) ;
#18872=DIRECTION ( 'NONE',  ( -0.9510565162951510887, -0.3090169943749553894, 0.000000000000000000 ) ) ;
#18882=ORIENTED_EDGE ( 'NONE', *, *, #6361, .T. ) ;
#18893=CARTESIAN_POINT ( 'NONE',  ( -160.0000000000000000, 0.000000000000000000, -100.0000000000000000 ) ) ;
#18896=DIRECTION ( 'NONE',  ( 1.000000000000000000, 0.000000000000000000, 0.000000000000000000 ) ) ;
#18910=CIRCLE ( 'NONE', #5430, 7.500000000000000888 ) ;
#18912=CARTESIAN_POINT ( 'NONE',  ( 0.000000000000000000, 0.000000000000000000, 100.0000000000000000 ) ) ;
#18913=DIRECTION ( 'NONE',  ( 1.000000000000000000, 0.000000000000000000, 0.000000000000000000 ) ) ;
#18915=ORIENTED_EDGE ( 'NONE', *, *, #2601, .T. ) ;
#18917=DIRECTION ( 'NONE',  ( -0.000000000000000000, -0.000000000000000000, -1.000000000000000000 ) ) ;
#18934=DIRECTION ( 'NONE',  ( -0.000000000000000000, -0.000000000000000000, 1.000000000000000000 ) ) ;
#18938=DIRECTION ( 'NONE',  ( 0.5877852522924826850, -0.8090169943749405679, 0.000000000000000000 ) ) ;
#18964=DIRECTION ( 'NONE',  ( 1.000000000000000000, 0.000000000000000000, 0.000000000000000000 ) ) ;
#18992=DIRECTION ( 'NONE',  ( 0.000000000000000000, 0.000000000000000000, 1.000000000000000000 ) ) ;
#19005=DIRECTION ( 'NONE',  ( 1.000000000000000000, 0.000000000000000000, 0.000000000000000000 ) ) ;
#19017=ORIENTED_EDGE ( 'NONE', *, *, #20454, .T. ) ;
#19018=DIRECTION ( 'NONE',  ( -1.000000000000000000, 0.000000000000000000, 0.000000000000000000 ) ) ;
#19045=CYLINDRICAL_SURFACE ( 'NONE', #11505, 145.0000000000000284 ) ;
#19046=DIRECTION ( 'NONE',  ( 1.000000000000000000, 0.000000000000000000, 0.000000000000000000 ) ) ;
#19056=ORIENTED_EDGE ( 'NONE', *, *, #23380, .F. ) ;
#19073=AXIS2_PLACEMENT_3D ( 'NONE', #23753, #14487, #5289 ) ;
#19085=EDGE_CURVE ( 'NONE', #20130, #7169, #22861, .T. ) ;
#19095=DIRECTION ( 'NONE',  ( 0.000000000000000000, 0.000000000000000000, 1.000000000000000000 ) ) ;
#19101=DIRECTION ( 'NONE',  ( 0.000000000000000000, 0.000000000000000000, 1.000000000000000000 ) ) ;
#19108=DIRECTION ( 'NONE',  ( -0.000000000000000000, -0.000000000000000000, 1.000000000000000000 ) ) ;
#19123=DIRECTION ( 'NONE',  ( 1.000000000000000000, 0.000000000000000000, 0.000000000000000000 ) ) ;
#19127=ORIENTED_EDGE ( 'NONE', *, *, #19927, .T. ) ;
#19128=DIRECTION ( 'NONE',  ( 1.000000000000000000, 0.000000000000000000, 0.000000000000000000 ) ) ;
#19135=VERTEX_POINT ( 'NONE', #16786 ) ;
#19143=( NAMED_UNIT ( * ) SI_UNIT ( $, .STERADIAN. ) SOLID_ANGLE_UNIT ( ) );
#19146=LINE ( 'NONE', #22890, #14765 ) ;
#19150=DIRECTION ( 'NONE',  ( -0.000000000000000000, 0.000000000000000000, -1.000000000000000000 ) ) ;
#19161=CARTESIAN_POINT ( 'NONE',  ( 0.000000000000000000, 0.000000000000000000, -90.00000000000000000 ) ) ;
#19179=AXIS2_PLACEMENT_3D ( 'NONE', #9284, #22054, #12696 ) ;
#19210=DIRECTION ( 'NONE',  ( 0.000000000000000000, -0.000000000000000000, 1.000000000000000000 ) ) ;
#19229=AXIS2_PLACEMENT_3D ( 'NONE', #19286, #4327, #11733 ) ;
#19237=DIRECTION ( 'NONE',  ( 0.000000000000000000, 0.000000000000000000, 1.000000000000000000 ) ) ;
#19240=CARTESIAN_POINT ( 'NONE',  ( -140.0355749532208449, -37.61698748598667663, -2.775557561562891351E-14 ) ) ;
#19244=VECTOR ( 'NONE', #20297, 1000.000000000000000 ) ;
#19247=ORIENTED_EDGE ( 'NONE', *, *, #2339, .T. ) ;
#19248=CIRCLE ( 'NONE', #3108, 7.500000000000003553 ) ;
#19261=FACE_OUTER_BOUND ( 'NONE', #23455, .T. ) ;
#19263=ORIENTED_EDGE ( 'NONE', *, *, #3305, .T. ) ;
#19273=DIRECTION ( 'NONE',  ( -0.9510565162951557516, 0.3090169943749406234, 0.000000000000000000 ) ) ;
#19278=CARTESIAN_POINT ( 'NONE',  ( -140.0355749532211007, 37.61698748598567477, -90.00000000000000000 ) ) ;
#19280=CYLINDRICAL_SURFACE ( 'NONE', #12550, 7.500000000000007105 ) ;
#19284=CARTESIAN_POINT ( 'NONE',  ( 37.61698748598715980, -140.0355749532207028, -2.775557561562891351E-14 ) ) ;
#19286=CARTESIAN_POINT ( 'NONE',  ( -117.3074641843669781, -85.22886158240918064, 90.00000000000000000 ) ) ;
#19294=CARTESIAN_POINT ( 'NONE',  ( 0.000000000000000000, 0.000000000000000000, -90.00000000000000000 ) ) ;
#19302=CARTESIAN_POINT ( 'NONE',  ( 7.497491405671719455, -144.8060344827586334, 90.00000000000000000 ) ) ;
#19316=ORIENTED_EDGE ( 'NONE', *, *, #1215, .F. ) ;
#19333=DIRECTION ( 'NONE',  ( -3.700743415417187942E-15, 1.000000000000000000, 0.000000000000000000 ) ) ;
#19350=CARTESIAN_POINT ( 'NONE',  ( -37.30746418436748968, 137.9031948627972781, 90.00000000000000000 ) ) ;
#19363=EDGE_CURVE ( 'NONE', #21483, #9371, #21214, .T. ) ;
#19365=ORIENTED_EDGE ( 'NONE', *, *, #11723, .F. ) ;
#19366=DIRECTION ( 'NONE',  ( 1.000000000000000000, 0.000000000000000000, 0.000000000000000000 ) ) ;
#19367=CARTESIAN_POINT ( 'NONE',  ( 85.22886158240706322, 117.3074641843685129, 90.00000000000000000 ) ) ;
#19369=CARTESIAN_POINT ( 'NONE',  ( 0.000000000000000000, 0.000000000000000000, 90.00000000000000000 ) ) ;
#19371=ORIENTED_EDGE ( 'NONE', *, *, #15942, .F. ) ;
#19390=CIRCLE ( 'NONE', #9002, 7.500000000000001776 ) ;
#19410=EDGE_LOOP ( 'NONE', ( #13533, #23669, #15964, #12835 ) ) ;
#19412=DIRECTION ( 'NONE',  ( 1.000000000000000000, 0.000000000000000000, 0.000000000000000000 ) ) ;
#19417=AXIS2_PLACEMENT_3D ( 'NONE', #14605, #1312, #10645 ) ;
#19430=AXIS2_PLACEMENT_3D ( 'NONE', #19367, #1009, #13748 ) ;
#19451=ORIENTED_EDGE ( 'NONE', *, *, #3633, .F. ) ;
#19455=DIRECTION ( 'NONE',  ( -1.000000000000000000, 0.000000000000000000, 0.000000000000000000 ) ) ;
#19468=ORIENTED_EDGE ( 'NONE', *, *, #6868, .T. ) ;
#19473=DIRECTION ( 'NONE',  ( 0.000000000000000000, 0.000000000000000000, 1.000000000000000000 ) ) ;
#19511=CYLINDRICAL_SURFACE ( 'NONE', #11120, 145.0000000000000284 ) ;
#19516=CARTESIAN_POINT ( 'NONE',  ( -85.22886158240879695, 117.3074641843673049, -90.00000000000000000 ) ) ;
#19517=ORIENTED_EDGE ( 'NONE', *, *, #20234, .T. ) ;
#19535=CARTESIAN_POINT ( 'NONE',  ( 0.000000000000000000, 0.000000000000000000, 90.00000000000000000 ) ) ;
#19538=ORIENTED_EDGE ( 'NONE', *, *, #22169, .T. ) ;
#19544=ORIENTED_EDGE ( 'NONE', *, *, #14939, .F. ) ;
#19553=ORIENTED_EDGE ( 'NONE', *, *, #17571, .T. ) ;
#19559=AXIS2_PLACEMENT_3D ( 'NONE', #22642, #8397, #2831 ) ;
#19570=ORIENTED_EDGE ( 'NONE', *, *, #20391, .F. ) ;
#19576=LINE ( 'NONE', #6434, #3475 ) ;
#19587=CIRCLE ( 'NONE', #13097, 145.0000000000000284 ) ;
#19606=AXIS2_PLACEMENT_3D ( 'NONE', #22277, #22156, #16497 ) ;
#19609=ORIENTED_EDGE ( 'NONE', *, *, #12705, .T. ) ;
#19644=DIRECTION ( 'NONE',  ( 1.000000000000000000, 0.000000000000000000, 0.000000000000000000 ) ) ;
#19649=DIRECTION ( 'NONE',  ( 1.000000000000000000, 0.000000000000000000, 0.000000000000000000 ) ) ;
#19656=AXIS2_PLACEMENT_3D ( 'NONE', #5263, #9011, #17709 ) ;
#19683=CARTESIAN_POINT ( 'NONE',  ( 0.000000000000000000, 145.0000000000000284, -90.00000000000000000 ) ) ;
#19702=ORIENTED_EDGE ( 'NONE', *, *, #1911, .F. ) ;
#19703=DIRECTION ( 'NONE',  ( 0.000000000000000000, 0.000000000000000000, 1.000000000000000000 ) ) ;
#19714=CARTESIAN_POINT ( 'NONE',  ( -37.61698748598514896, -140.0355749532212428, 90.00000000000000000 ) ) ;
#19720=ORIENTED_EDGE ( 'NONE', *, *, #16990, .T. ) ;
#19721=CYLINDRICAL_SURFACE ( 'NONE', #21772, 7.500000000000000000 ) ;
#19753=VERTEX_POINT ( 'NONE', #16150 ) ;
#19789=CARTESIAN_POINT ( 'NONE',  ( 0.000000000000000000, 145.0000000000000284, 90.00000000000000000 ) ) ;
#19791=FACE_BOUND ( 'NONE', #3075, .T. ) ;
#19793=CIRCLE ( 'NONE', #5520, 7.500000000000006217 ) ;
#19817=MANIFOLD_SOLID_BREP ( 'Cut-Extrude-Thin2', #10257 ) ;
#19832=EDGE_CURVE ( 'NONE', #22779, #10209, #8120, .T. ) ;
#19833=VERTEX_POINT ( 'NONE', #3670 ) ;
#19846=CARTESIAN_POINT ( 'NONE',  ( 0.000000000000000000, 0.000000000000000000, 100.0000000000000000 ) ) ;
#19860=EDGE_LOOP ( 'NONE', ( #22360, #19570, #2645, #15222 ) ) ;
#19873=DIRECTION ( 'NONE',  ( -0.000000000000000000, 1.000000000000000000, 0.000000000000000000 ) ) ;
#19875=VERTEX_POINT ( 'NONE', #18893 ) ;
#19893=ADVANCED_FACE ( 'NONE', ( #11575 ), #11446, .T. ) ;
#19895=ORIENTED_EDGE ( 'NONE', *, *, #11687, .T. ) ;
#19913=DIRECTION ( 'NONE',  ( -0.000000000000000000, -0.000000000000000000, 1.000000000000000000 ) ) ;
#19927=EDGE_CURVE ( 'NONE', #13438, #21770, #6228, .T. ) ;
#19929=EDGE_CURVE ( 'NONE', #3142, #8675, #22767, .T. ) ;
#19931=AXIS2_PLACEMENT_3D ( 'NONE', #15955, #14161, #21490 ) ;
#19943=DIRECTION ( 'NONE',  ( 1.000000000000000000, 0.000000000000000000, 0.000000000000000000 ) ) ;
#19947=CIRCLE ( 'NONE', #2202, 7.500000000000000888 ) ;
#19967=DIRECTION ( 'NONE',  ( 1.000000000000000000, 0.000000000000000000, 0.000000000000000000 ) ) ;
#19985=CARTESIAN_POINT ( 'NONE',  ( 7.499999999999999112, 0.000000000000000000, 100.0000000000000000 ) ) ;
#19991=LINE ( 'NONE', #3796, #1083 ) ;
#19999=ORIENTED_EDGE ( 'NONE', *, *, #14592, .F. ) ;
#20003=PRODUCT ( 'head pulley', 'head pulley', '', ( #21099 ) ) ;
#20018=ORIENTED_EDGE ( 'NONE', *, *, #3031, .T. ) ;
#20037=ADVANCED_FACE ( 'NONE', ( #1259 ), #21421, .F. ) ;
#20053=CARTESIAN_POINT ( 'NONE',  ( -137.9031948627974486, 44.80746418436699940, -90.00000000000000000 ) ) ;
#20073=EDGE_CURVE ( 'NONE', #11805, #10493, #10585, .T. ) ;
#20079=VERTEX_POINT ( 'NONE', #1141 ) ;
#20086=CARTESIAN_POINT ( 'NONE',  ( -160.0000000000000000, 0.000000000000000000, -90.00000000000000000 ) ) ;
#20100=CARTESIAN_POINT ( 'NONE',  ( 91.18044947428789726, 112.7436279071541776, -90.00000000000000000 ) ) ;
#20105=EDGE_CURVE ( 'NONE', #23533, #20130, #13109, .T. ) ;
#20112=DIRECTION ( 'NONE',  ( 0.000000000000000000, 0.000000000000000000, 1.000000000000000000 ) ) ;
#20127=ORIENTED_EDGE ( 'NONE', *, *, #3883, .F. ) ;
#20130=VERTEX_POINT ( 'NONE', #5357 ) ;
#20134=ORIENTED_EDGE ( 'NONE', *, *, #835, .F. ) ;
#20139=VERTEX_POINT ( 'NONE', #14437 ) ;
#20140=ORIENTED_EDGE ( 'NONE', *, *, #2157, .F. ) ;
#20152=LINE ( 'NONE', #21738, #14924 ) ;
#20153=ORIENTED_EDGE ( 'NONE', *, *, #10315, .F. ) ;
#20157=EDGE_CURVE ( 'NONE', #10526, #20363, #10404, .T. ) ;
#20198=SHAPE_REPRESENTATION_RELATIONSHIP ( 'NONE' , 'NONE' ,  #8847, #11926 ) ;
#20204=ORIENTED_EDGE ( 'NONE', *, *, #9417, .T. ) ;
#20220=( NAMED_UNIT ( * ) SI_UNIT ( $, .STERADIAN. ) SOLID_ANGLE_UNIT ( ) );
#20230=EDGE_CURVE ( 'NONE', #5086, #19875, #14909, .T. ) ;
#20234=EDGE_CURVE ( 'NONE', #3110, #22784, #4000, .T. ) ;
#20237=VECTOR ( 'NONE', #1791, 1000.000000000000000 ) ;
#20251=ORIENTED_EDGE ( 'NONE', *, *, #13547, .F. ) ;
#20255=DIRECTION ( 'NONE',  ( 1.000000000000000000, 0.000000000000000000, 0.000000000000000000 ) ) ;
#20261=AXIS2_PLACEMENT_3D ( 'NONE', #1278, #1032, #2745 ) ;
#20265=CIRCLE ( 'NONE', #21812, 35.00000000000000711 ) ;
#20267=LINE ( 'NONE', #9186, #5296 ) ;
#20274=VERTEX_POINT ( 'NONE', #20440 ) ;
#20289=CARTESIAN_POINT ( 'NONE',  ( -144.8060344827586050, -7.497491405672224829, -90.00000000000000000 ) ) ;
#20297=DIRECTION ( 'NONE',  ( 0.000000000000000000, 0.000000000000000000, -1.000000000000000000 ) ) ;
#20304=DIRECTION ( 'NONE',  ( 0.000000000000000000, 0.000000000000000000, 1.000000000000000000 ) ) ;
#20305=CARTESIAN_POINT ( 'NONE',  ( -79.04925354955248906, 121.5574576620396812, -2.775557561562891351E-14 ) ) ;
#20336=CARTESIAN_POINT ( 'NONE',  ( 91.18044947429038416, -112.7436279071521881, -90.00000000000000000 ) ) ;
#20344=VERTEX_POINT ( 'NONE', #17785 ) ;
#20347=ORIENTED_EDGE ( 'NONE', *, *, #6630, .F. ) ;
#20363=VERTEX_POINT ( 'NONE', #17425 ) ;
#20379=CARTESIAN_POINT ( 'NONE',  ( 140.0355749532213565, -37.61698748598472974, -2.775557561562891351E-14 ) ) ;
#20386=ORIENTED_EDGE ( 'NONE', *, *, #13051, .T. ) ;
#20387=DIRECTION ( 'NONE',  ( 1.000000000000000000, 0.000000000000000000, 0.000000000000000000 ) ) ;
#20390=CIRCLE ( 'NONE', #13131, 7.500000000000000888 ) ;
#20391=EDGE_CURVE ( 'NONE', #4114, #23301, #9572, .T. ) ;
#20395=CIRCLE ( 'NONE', #16617, 145.0000000000000284 ) ;
#20420=( GEOMETRIC_REPRESENTATION_CONTEXT ( 3 ) GLOBAL_UNCERTAINTY_ASSIGNED_CONTEXT ( ( #17422 ) ) GLOBAL_UNIT_ASSIGNED_CONTEXT ( ( #16356, #10948, #19143 ) ) REPRESENTATION_CONTEXT ( 'NONE', 'WORKASPACE' ) );
#20429=ADVANCED_FACE ( 'NONE', ( #8140 ), #17527, .T. ) ;
#20440=CARTESIAN_POINT ( 'NONE',  ( -121.5574576620394112, -79.04925354955290118, -90.00000000000000000 ) ) ;
#20444=DIRECTION ( 'NONE',  ( 0.000000000000000000, 0.000000000000000000, 1.000000000000000000 ) ) ;
#20454=EDGE_CURVE ( 'NONE', #10981, #2765, #6479, .T. ) ;
#20501=EDGE_CURVE ( 'NONE', #12981, #19833, #8044, .T. ) ;
#20538=ORIENTED_EDGE ( 'NONE', *, *, #14524, .T. ) ;
#20547=ORIENTED_EDGE ( 'NONE', *, *, #11016, .T. ) ;
#20550=CARTESIAN_POINT ( 'NONE',  ( -130.4031948627974486, 44.80746418436699940, -90.00000000000000000 ) ) ;
#20570=DIRECTION ( 'NONE',  ( 0.000000000000000000, 0.000000000000000000, 1.000000000000000000 ) ) ;
#20584=ORIENTED_EDGE ( 'NONE', *, *, #2033, .F. ) ;
#20591=DIRECTION ( 'NONE',  ( 1.000000000000000000, 0.000000000000000000, 0.000000000000000000 ) ) ;
#20615=CYLINDRICAL_SURFACE ( 'NONE', #8703, 145.0000000000000284 ) ;
#20620=EDGE_CURVE ( 'NONE', #766, #11911, #3735, .T. ) ;
#20626=DIRECTION ( 'NONE',  ( 0.000000000000000000, 0.000000000000000000, 1.000000000000000000 ) ) ;
#20628=CIRCLE ( 'NONE', #18689, 145.0000000000000284 ) ;
#20631=DIRECTION ( 'NONE',  ( 1.000000000000000000, 0.000000000000000000, 0.000000000000000000 ) ) ;
#20663=ORIENTED_EDGE ( 'NONE', *, *, #4109, .F. ) ;
#20679=CARTESIAN_POINT ( 'NONE',  ( 0.000000000000000000, 0.000000000000000000, -90.00000000000000000 ) ) ;
#20711=AXIS2_PLACEMENT_3D ( 'NONE', #9537, #13207, #22321 ) ;
#20714=ORIENTED_EDGE ( 'NONE', *, *, #22555, .T. ) ;
#20716=CARTESIAN_POINT ( 'NONE',  ( -37.61698748598617215, 140.0355749532209586, -90.00000000000000000 ) ) ;
#20721=LINE ( 'NONE', #811, #10532 ) ;
#20723=DIRECTION ( 'NONE',  ( 1.000000000000000000, 0.000000000000000000, 0.000000000000000000 ) ) ;
#20758=MECHANICAL_DESIGN_GEOMETRIC_PRESENTATION_REPRESENTATION('',(#10770),#14627);
#20760=AXIS2_PLACEMENT_3D ( 'NONE', #18642, #4165, #9501 ) ;
#20778=AXIS2_PLACEMENT_3D ( 'NONE', #10704, #20304, #13003 ) ;
#20783=AXIS2_PLACEMENT_3D ( 'NONE', #17575, #909, #1389 ) ;
#20828=EDGE_LOOP ( 'NONE', ( #20901, #14968, #15708, #7352 ) ) ;
#20841=CYLINDRICAL_SURFACE ( 'NONE', #569, 7.500000000000007105 ) ;
#20901=ORIENTED_EDGE ( 'NONE', *, *, #19832, .F. ) ;
#20930=DIRECTION ( 'NONE',  ( 0.000000000000000000, 0.000000000000000000, 1.000000000000000000 ) ) ;
#20936=CARTESIAN_POINT ( 'NONE',  ( 0.000000000000000000, 0.000000000000000000, -100.0000000000000000 ) ) ;
#20939=EDGE_CURVE ( 'NONE', #22438, #11911, #7644, .T. ) ;
#20946=ORIENTED_EDGE ( 'NONE', *, *, #13058, .T. ) ;
#20962=CARTESIAN_POINT ( 'NONE',  ( -121.5574576620399654, 79.04925354955206274, -2.775557561562891351E-14 ) ) ;
#20965=DIRECTION ( 'NONE',  ( 1.000000000000000000, 0.000000000000000000, -0.000000000000000000 ) ) ;
#20970=ORIENTED_EDGE ( 'NONE', *, *, #17571, .F. ) ;
#20986=EDGE_CURVE ( 'NONE', #8126, #9666, #15770, .T. ) ;
#21033=UNCERTAINTY_MEASURE_WITH_UNIT (LENGTH_MEASURE( 1.000000000000000082E-05 ), #2083, 'distance_accuracy_value', 'NONE');
#21047=CARTESIAN_POINT ( 'NONE',  ( 51.87806360044629628, 135.4018704341563364, 90.00000000000000000 ) ) ;
#21061=CARTESIAN_POINT ( 'NONE',  ( -51.87806360044717735, -135.4018704341559669, -2.775557561562891351E-14 ) ) ;
#21071=EDGE_CURVE ( 'NONE', #13072, #17463, #11960, .T. ) ;
#21088=CARTESIAN_POINT ( 'NONE',  ( -44.80746418436648071, -137.9031948627975908, 90.00000000000000000 ) ) ;
#21089=DIRECTION ( 'NONE',  ( 1.000000000000000000, 0.000000000000000000, 0.000000000000000000 ) ) ;
#21094=FACE_OUTER_BOUND ( 'NONE', #18416, .T. ) ;
#21099=PRODUCT_CONTEXT ( 'NONE', #8923, 'mechanical' ) ;
#21108=LINE ( 'NONE', #4567, #23116 ) ;
#21111=ADVANCED_FACE ( 'NONE', ( #13749 ), #6342, .T. ) ;
#21150=CYLINDRICAL_SURFACE ( 'NONE', #4427, 7.500000000000007105 ) ;
#21163=VECTOR ( 'NONE', #7671, 1000.000000000000000 ) ;
#21186=ORIENTED_EDGE ( 'NONE', *, *, #20157, .T. ) ;
#21188=LINE ( 'NONE', #15537, #6377 ) ;
#21192=VECTOR ( 'NONE', #3267, 1000.000000000000000 ) ;
#21214=CIRCLE ( 'NONE', #261, 145.0000000000000284 ) ;
#21223=ORIENTED_EDGE ( 'NONE', *, *, #20986, .T. ) ;
#21225=DIRECTION ( 'NONE',  ( -0.8090169943749428993, -0.5877852522924793544, 0.000000000000000000 ) ) ;
#21236=DIRECTION ( 'NONE',  ( -0.000000000000000000, -0.000000000000000000, 1.000000000000000000 ) ) ;
#21253=EDGE_CURVE ( 'NONE', #18161, #11805, #6817, .T. ) ;
#21255=ORIENTED_EDGE ( 'NONE', *, *, #12059, .F. ) ;
#21272=DIRECTION ( 'NONE',  ( 1.000000000000000000, 0.000000000000000000, 0.000000000000000000 ) ) ;
#21284=EDGE_CURVE ( 'NONE', #3693, #11696, #7287, .T. ) ;
#21287=DIRECTION ( 'NONE',  ( 1.000000000000000000, 0.000000000000000000, 0.000000000000000000 ) ) ;
#21295=DIRECTION ( 'NONE',  ( -0.000000000000000000, -0.000000000000000000, 1.000000000000000000 ) ) ;
#21305=VERTEX_POINT ( 'NONE', #8996 ) ;
#21317=VERTEX_POINT ( 'NONE', #14793 ) ;
#21353=EDGE_LOOP ( 'NONE', ( #5181, #5569, #6546, #19247 ) ) ;
#21385=DIRECTION ( 'NONE',  ( -0.000000000000000000, -0.000000000000000000, 1.000000000000000000 ) ) ;
#21386=DIRECTION ( 'NONE',  ( -0.000000000000000000, -0.000000000000000000, 1.000000000000000000 ) ) ;
#21392=CARTESIAN_POINT ( 'NONE',  ( 0.000000000000000000, 0.000000000000000000, -90.00000000000000000 ) ) ;
#21395=VERTEX_POINT ( 'NONE', #19302 ) ;
#21410=EDGE_CURVE ( 'NONE', #9726, #20363, #23497, .T. ) ;
#21421=CYLINDRICAL_SURFACE ( 'NONE', #15788, 7.500000000000007105 ) ;
#21449=CYLINDRICAL_SURFACE ( 'NONE', #20261, 145.0000000000000284 ) ;
#21451=DIRECTION ( 'NONE',  ( 0.000000000000000000, 0.000000000000000000, 1.000000000000000000 ) ) ;
#21460=ORIENTED_EDGE ( 'NONE', *, *, #22440, .F. ) ;
#21462=CARTESIAN_POINT ( 'NONE',  ( -85.22886158240879695, 117.3074641843673049, 90.00000000000000000 ) ) ;
#21464=DIRECTION ( 'NONE',  ( 0.000000000000000000, 0.000000000000000000, 1.000000000000000000 ) ) ;
#21465=EDGE_LOOP ( 'NONE', ( #14775, #14417, #3587, #15667 ) ) ;
#21470=ORIENTED_EDGE ( 'NONE', *, *, #17834, .F. ) ;
#21476=AXIS2_PLACEMENT_3D ( 'NONE', #19683, #1323, #23052 ) ;
#21483=VERTEX_POINT ( 'NONE', #22843 ) ;
#21490=DIRECTION ( 'NONE',  ( 1.000000000000000000, 0.000000000000000000, 0.000000000000000000 ) ) ;
#21491=ORIENTED_EDGE ( 'NONE', *, *, #5924, .T. ) ;
#21509=CARTESIAN_POINT ( 'NONE',  ( 0.000000000000000000, 0.000000000000000000, -90.00000000000000000 ) ) ;
#21535=CARTESIAN_POINT ( 'NONE',  ( -121.5574576620399654, 79.04925354955206274, -90.00000000000000000 ) ) ;
#21555=EDGE_CURVE ( 'NONE', #11696, #17056, #23086, .T. ) ;
#21557=PRODUCT_DEFINITION ( 'UNKNOWN', '', #9275, #16773 ) ;
#21560=CYLINDRICAL_SURFACE ( 'NONE', #15842, 145.0000000000000284 ) ;
#21564=EDGE_LOOP ( 'NONE', ( #5293, #21491, #11671, #20970 ) ) ;
#21569=CARTESIAN_POINT ( 'NONE',  ( 0.000000000000000000, 0.000000000000000000, -90.00000000000000000 ) ) ;
#21576=FACE_OUTER_BOUND ( 'NONE', #17395, .T. ) ;
#21592=ORIENTED_EDGE ( 'NONE', *, *, #19363, .F. ) ;
#21593=EDGE_CURVE ( 'NONE', #2320, #23165, #1513, .T. ) ;
#21642=DIRECTION ( 'NONE',  ( 1.000000000000000000, 0.000000000000000000, 0.000000000000000000 ) ) ;
#21661=ORIENTED_EDGE ( 'NONE', *, *, #2944, .T. ) ;
#21672=VERTEX_POINT ( 'NONE', #10920 ) ;
#21676=FACE_OUTER_BOUND ( 'NONE', #6420, .T. ) ;
#21681=ADVANCED_FACE ( 'NONE', ( #12625 ), #16567, .T. ) ;
#21685=DIRECTION ( 'NONE',  ( -0.000000000000000000, 0.000000000000000000, 1.000000000000000000 ) ) ;
#21688=FACE_OUTER_BOUND ( 'NONE', #17723, .T. ) ;
#21738=CARTESIAN_POINT ( 'NONE',  ( 112.7436279071538792, -91.18044947428830937, -2.775557561562891351E-14 ) ) ;
#21742=ORIENTED_EDGE ( 'NONE', *, *, #18454, .T. ) ;
#21752=DIRECTION ( 'NONE',  ( 0.000000000000000000, 0.000000000000000000, 1.000000000000000000 ) ) ;
#21768=DIRECTION ( 'NONE',  ( 1.000000000000000000, 0.000000000000000000, 0.000000000000000000 ) ) ;
#21770=VERTEX_POINT ( 'NONE', #18828 ) ;
#21772=AXIS2_PLACEMENT_3D ( 'NONE', #1368, #15890, #6808 ) ;
#21782=DIRECTION ( 'NONE',  ( 1.000000000000000000, 0.000000000000000000, 0.000000000000000000 ) ) ;
#21812=AXIS2_PLACEMENT_3D ( 'NONE', #19846, #19473, #1004 ) ;
#21813=ORIENTED_EDGE ( 'NONE', *, *, #15508, .T. ) ;
#21823=CARTESIAN_POINT ( 'NONE',  ( -130.4031948627971076, -44.80746418436799416, 90.00000000000000000 ) ) ;
#21830=ORIENTED_EDGE ( 'NONE', *, *, #18138, .F. ) ;
#21836=CYLINDRICAL_SURFACE ( 'NONE', #10556, 7.500000000000007105 ) ;
#21837=EDGE_CURVE ( 'NONE', #17692, #23165, #16477, .T. ) ;
#21858=DIRECTION ( 'NONE',  ( 0.000000000000000000, 0.000000000000000000, 1.000000000000000000 ) ) ;
#21863=AXIS2_PLACEMENT_3D ( 'NONE', #16919, #9295, #16301 ) ;
#21886=DIRECTION ( 'NONE',  ( 0.3090169943749589421, -0.9510565162951498674, 0.000000000000000000 ) ) ;
#21897=CIRCLE ( 'NONE', #14983, 145.0000000000000284 ) ;
#21922=ADVANCED_FACE ( 'NONE', ( #14845 ), #14490, .F. ) ;
#21931=VECTOR ( 'NONE', #18637, 1000.000000000000000 ) ;
#21936=VECTOR ( 'NONE', #6600, 1000.000000000000000 ) ;
#21958=AXIS2_PLACEMENT_3D ( 'NONE', #19369, #15185, #7920 ) ;
#21959=FACE_OUTER_BOUND ( 'NONE', #13077, .T. ) ;
#21988=DIRECTION ( 'NONE',  ( 0.000000000000000000, 0.000000000000000000, 1.000000000000000000 ) ) ;
#22018=LINE ( 'NONE', #20305, #7647 ) ;
#22019=DIRECTION ( 'NONE',  ( 0.9510565162951580831, -0.3090169943749334069, 0.000000000000000000 ) ) ;
#22025=DIRECTION ( 'NONE',  ( 0.000000000000000000, 0.000000000000000000, 1.000000000000000000 ) ) ;
#22028=CARTESIAN_POINT ( 'NONE',  ( 135.4018704341550574, 51.87806360044960741, 90.00000000000000000 ) ) ;
#22036=DIRECTION ( 'NONE',  ( 0.000000000000000000, 0.000000000000000000, 1.000000000000000000 ) ) ;
#22038=ADVANCED_FACE ( 'NONE', ( #17955 ), #19511, .T. ) ;
#22040=ORIENTED_EDGE ( 'NONE', *, *, #1762, .T. ) ;
#22054=DIRECTION ( 'NONE',  ( -0.000000000000000000, -0.000000000000000000, 1.000000000000000000 ) ) ;
#22058=ORIENTED_EDGE ( 'NONE', *, *, #3633, .T. ) ;
#22077=DIRECTION ( 'NONE',  ( -0.000000000000000000, -0.000000000000000000, 1.000000000000000000 ) ) ;
#22147=DIRECTION ( 'NONE',  ( 1.110223024625156383E-14, -1.000000000000000000, 0.000000000000000000 ) ) ;
#22156=DIRECTION ( 'NONE',  ( 0.000000000000000000, 0.000000000000000000, 1.000000000000000000 ) ) ;
#22158=ORIENTED_EDGE ( 'NONE', *, *, #3849, .T. ) ;
#22169=EDGE_CURVE ( 'NONE', #13199, #17672, #19991, .T. ) ;
#22183=AXIS2_PLACEMENT_3D ( 'NONE', #10039, #15699, #17392 ) ;
#22186=FACE_OUTER_BOUND ( 'NONE', #21353, .T. ) ;
#22194=EDGE_LOOP ( 'NONE', ( #7145, #21460, #12216, #16634 ) ) ;
#22251=CARTESIAN_POINT ( 'NONE',  ( 145.0000000000000284, 1.518794382396763073E-12, -90.00000000000000000 ) ) ;
#22259=EDGE_CURVE ( 'NONE', #3693, #10547, #21897, .T. ) ;
#22277=CARTESIAN_POINT ( 'NONE',  ( 0.000000000000000000, 0.000000000000000000, -90.00000000000000000 ) ) ;
#22286=CARTESIAN_POINT ( 'NONE',  ( -137.9031948627974486, 44.80746418436699940, -90.00000000000000000 ) ) ;
#22296=EDGE_LOOP ( 'NONE', ( #10451, #6014, #22560, #772, #18778, #12007, #3517, #18657, #1402, #11856, #4287, #22973, #12215, #1251, #5586, #22040, #14962, #2947, #2081, #8138, #17216, #22467, #3524, #19702, #450, #18218, #6173, #15367, #8627, #8252, #10329, #89, #13930, #7490, #1486, #18320, #16943, #17292, #13268, #16391, #14275, #4539, #12707, #9103, #8317, #12993, #19017, #11084, #21830 ) ) ;
#22312=AXIS2_PLACEMENT_3D ( 'NONE', #18775, #6351, #20591 ) ;
#22315=AXIS2_PLACEMENT_3D ( 'NONE', #19161, #10018, #1047 ) ;
#22321=DIRECTION ( 'NONE',  ( 0.5877852522924719159, 0.8090169943749482284, 0.000000000000000000 ) ) ;
#22328=AXIS2_PLACEMENT_3D ( 'NONE', #7640, #19101, #9954 ) ;
#22329=CIRCLE ( 'NONE', #1883, 35.00000000000000711 ) ;
#22331=CIRCLE ( 'NONE', #21958, 145.0000000000000284 ) ;
#22360=ORIENTED_EDGE ( 'NONE', *, *, #14684, .F. ) ;
#22362=CIRCLE ( 'NONE', #12790, 7.499999999999996447 ) ;
#22371=CIRCLE ( 'NONE', #22312, 145.0000000000000284 ) ;
#22380=( NAMED_UNIT ( * ) SI_UNIT ( $, .STERADIAN. ) SOLID_ANGLE_UNIT ( ) );
#22390=CARTESIAN_POINT ( 'NONE',  ( -7.499999999999999112, 0.000000000000000000, 100.0000000000000000 ) ) ;
#22416=FACE_OUTER_BOUND ( 'NONE', #22487, .T. ) ;
#22438=VERTEX_POINT ( 'NONE', #6455 ) ;
#22440=EDGE_CURVE ( 'NONE', #20130, #23533, #1456, .T. ) ;
#22445=ADVANCED_FACE ( 'NONE', ( #17926 ), #14095, .F. ) ;
#22451=ORIENTED_EDGE ( 'NONE', *, *, #9929, .T. ) ;
#22464=ORIENTED_EDGE ( 'NONE', *, *, #14638, .T. ) ;
#22467=ORIENTED_EDGE ( 'NONE', *, *, #3883, .T. ) ;
#22472=EDGE_CURVE ( 'NONE', #13321, #10981, #23117, .T. ) ;
#22476=CYLINDRICAL_SURFACE ( 'NONE', #7291, 7.500000000000007105 ) ;
#22485=CARTESIAN_POINT ( 'NONE',  ( 140.0355749532213281, -37.61698748598472264, -90.00000000000000000 ) ) ;
#22486=CARTESIAN_POINT ( 'NONE',  ( -77.72886158240878274, 117.3074641843673049, -90.00000000000000000 ) ) ;
#22487=EDGE_LOOP ( 'NONE', ( #21470, #19895, #15499, #20547 ) ) ;
#22523=VERTEX_POINT ( 'NONE', #10474 ) ;
#22524=DIRECTION ( 'NONE',  ( -0.000000000000000000, -0.000000000000000000, 1.000000000000000000 ) ) ;
#22526=CIRCLE ( 'NONE', #5554, 7.500000000000000000 ) ;
#22532=ADVANCED_FACE ( 'NONE', ( #6815 ), #12650, .F. ) ;
#22553=ORIENTED_EDGE ( 'NONE', *, *, #7064, .F. ) ;
#22555=EDGE_CURVE ( 'NONE', #22523, #2480, #22018, .T. ) ;
#22557=ORIENTED_EDGE ( 'NONE', *, *, #13607, .T. ) ;
#22560=ORIENTED_EDGE ( 'NONE', *, *, #18029, .F. ) ;
#22561=DIRECTION ( 'NONE',  ( 0.000000000000000000, 0.000000000000000000, 1.000000000000000000 ) ) ;
#22577=EDGE_LOOP ( 'NONE', ( #5336, #13489, #2720, #2303 ) ) ;
#22603=EDGE_CURVE ( 'NONE', #20079, #9726, #12786, .T. ) ;
#22626=EDGE_CURVE ( 'NONE', #14720, #13931, #3897, .T. ) ;
#22642=CARTESIAN_POINT ( 'NONE',  ( 0.000000000000000000, 0.000000000000000000, -100.0000000000000000 ) ) ;
#22648=DIRECTION ( 'NONE',  ( -0.000000000000000000, -0.000000000000000000, -1.000000000000000000 ) ) ;
#22684=ORIENTED_EDGE ( 'NONE', *, *, #6868, .F. ) ;
#22701=ORIENTED_EDGE ( 'NONE', *, *, #22603, .T. ) ;
#22709=ORIENTED_EDGE ( 'NONE', *, *, #12074, .T. ) ;
#22719=EDGE_LOOP ( 'NONE', ( #11369, #10294, #19609, #5759 ) ) ;
#22752=ADVANCED_FACE ( 'NONE', ( #4001 ), #2191, .T. ) ;
#22755=AXIS2_PLACEMENT_3D ( 'NONE', #9840, #4275, #11199 ) ;
#22757=EDGE_LOOP ( 'NONE', ( #533, #13839, #14568, #17261 ) ) ;
#22764=VERTEX_POINT ( 'NONE', #22485 ) ;
#22766=ORIENTED_EDGE ( 'NONE', *, *, #16077, .F. ) ;
#22767=LINE ( 'NONE', #7548, #21931 ) ;
#22779=VERTEX_POINT ( 'NONE', #12120 ) ;
#22784=VERTEX_POINT ( 'NONE', #2877 ) ;
#22786=DIRECTION ( 'NONE',  ( 1.000000000000000000, 0.000000000000000000, 0.000000000000000000 ) ) ;
#22819=ORIENTED_EDGE ( 'NONE', *, *, #7650, .F. ) ;
#22830=DIRECTION ( 'NONE',  ( 0.000000000000000000, 0.000000000000000000, 1.000000000000000000 ) ) ;
#22836=DIRECTION ( 'NONE',  ( -0.000000000000000000, -0.000000000000000000, 1.000000000000000000 ) ) ;
#22843=CARTESIAN_POINT ( 'NONE',  ( 51.87806360044913134, -135.4018704341552564, -90.00000000000000000 ) ) ;
#22848=DIRECTION ( 'NONE',  ( 0.000000000000000000, 0.000000000000000000, 1.000000000000000000 ) ) ;
#22861=LINE ( 'NONE', #13983, #11594 ) ;
#22869=CARTESIAN_POINT ( 'NONE',  ( 0.000000000000000000, 0.000000000000000000, 90.00000000000000000 ) ) ;
#22878=ADVANCED_FACE ( 'NONE', ( #19791, #21959 ), #12715, .T. ) ;
#22885=DIRECTION ( 'NONE',  ( 1.000000000000000000, 0.000000000000000000, 0.000000000000000000 ) ) ;
#22890=CARTESIAN_POINT ( 'NONE',  ( -140.0355749532211007, 37.61698748598567477, -2.775557561562891351E-14 ) ) ;
#22892=ORIENTED_EDGE ( 'NONE', *, *, #2575, .F. ) ;
#22902=VECTOR ( 'NONE', #6839, 1000.000000000000000 ) ;
#22915=AXIS2_PLACEMENT_3D ( 'NONE', #11684, #16970, #15167 ) ;
#22936=AXIS2_PLACEMENT_3D ( 'NONE', #10527, #12003, #2990 ) ;
#22948=UNCERTAINTY_MEASURE_WITH_UNIT (LENGTH_MEASURE( 1.000000000000000082E-05 ), #10972, 'distance_accuracy_value', 'NONE');
#22951=CARTESIAN_POINT ( 'NONE',  ( -137.9031948627971076, -44.80746418436799416, -90.00000000000000000 ) ) ;
#22964=AXIS2_PLACEMENT_3D ( 'NONE', #1741, #22036, #22147 ) ;
#22973=ORIENTED_EDGE ( 'NONE', *, *, #14624, .F. ) ;
#22978=EDGE_LOOP ( 'NONE', ( #16902, #5910, #2509, #20584, #1085, #13108, #7084, #19553, #20251, #4997, #16823, #11533, #4260, #13378, #18488, #5964, #10025, #23680, #10983, #23752, #16785, #10201, #12498, #23420, #21592, #10247, #923, #18531, #19056, #8508, #12065, #16338, #19468, #12113, #5811, #18882, #3877, #14363, #15703, #114, #4924, #16771, #18915, #14151, #23224, #8469, #7863, #17909, #7661 ) ) ;
#23002=CARTESIAN_POINT ( 'NONE',  ( -77.72886158240795851, -117.3074641843678876, -90.00000000000000000 ) ) ;
#23026=ADVANCED_FACE ( 'NONE', ( #5790, #5656 ), #2258, .T. ) ;
#23028=ORIENTED_EDGE ( 'NONE', *, *, #21837, .T. ) ;
#23048=CIRCLE ( 'NONE', #7226, 145.0000000000000284 ) ;
#23049=DIRECTION ( 'NONE',  ( -0.000000000000000000, -0.000000000000000000, 1.000000000000000000 ) ) ;
#23052=DIRECTION ( 'NONE',  ( 1.000000000000000000, 0.000000000000000000, 0.000000000000000000 ) ) ;
#23053=AXIS2_PLACEMENT_3D ( 'NONE', #21088, #11962, #19273 ) ;
#23062=DIRECTION ( 'NONE',  ( -0.5877852522924773560, 0.8090169943749444537, 0.000000000000000000 ) ) ;
#23073=AXIS2_PLACEMENT_3D ( 'NONE', #1229, #7136, #12263 ) ;
#23081=EDGE_LOOP ( 'NONE', ( #19517, #2919, #23127, #7440 ) ) ;
#23086=CIRCLE ( 'NONE', #2670, 145.0000000000000284 ) ;
#23089=CARTESIAN_POINT ( 'NONE',  ( 0.000000000000000000, -145.0000000000000284, 90.00000000000000000 ) ) ;
#23116=VECTOR ( 'NONE', #1541, 1000.000000000000000 ) ;
#23117=LINE ( 'NONE', #3070, #2230 ) ;
#23120=DIRECTION ( 'NONE',  ( 0.000000000000000000, 0.000000000000000000, 1.000000000000000000 ) ) ;
#23127=ORIENTED_EDGE ( 'NONE', *, *, #11514, .T. ) ;
#23165=VERTEX_POINT ( 'NONE', #2852 ) ;
#23168=ORIENTED_EDGE ( 'NONE', *, *, #6633, .T. ) ;
#23184=ORIENTED_EDGE ( 'NONE', *, *, #10844, .T. ) ;
#23189=EDGE_CURVE ( 'NONE', #9666, #14205, #8838, .T. ) ;
#23202=DIRECTION ( 'NONE',  ( 1.000000000000000000, 0.000000000000000000, 0.000000000000000000 ) ) ;
#23208=EDGE_CURVE ( 'NONE', #22764, #16743, #13887, .T. ) ;
#23224=ORIENTED_EDGE ( 'NONE', *, *, #6770, .T. ) ;
#23229=CARTESIAN_POINT ( 'NONE',  ( -137.9031948627971076, -44.80746418436799416, -90.00000000000000000 ) ) ;
#23237=FACE_OUTER_BOUND ( 'NONE', #16018, .T. ) ;
#23239=ORIENTED_EDGE ( 'NONE', *, *, #15235, .T. ) ;
#23268=VECTOR ( 'NONE', #12358, 1000.000000000000000 ) ;
#23300=ADVANCED_FACE ( 'NONE', ( #23389, #23625 ), #23516, .F. ) ;
#23301=VERTEX_POINT ( 'NONE', #7082 ) ;
#23340=CARTESIAN_POINT ( 'NONE',  ( -7.499999999999999112, 41.99999999999998579, 100.0000000000000000 ) ) ;
#23380=EDGE_CURVE ( 'NONE', #12572, #15709, #5368, .T. ) ;
#23381=CARTESIAN_POINT ( 'NONE',  ( 140.0355749532205891, 37.61698748598766429, -2.775557561562891351E-14 ) ) ;
#23389=FACE_BOUND ( 'NONE', #22296, .T. ) ;
#23393=DIRECTION ( 'NONE',  ( 0.000000000000000000, -0.000000000000000000, 1.000000000000000000 ) ) ;
#23420=ORIENTED_EDGE ( 'NONE', *, *, #1307, .T. ) ;
#23427=ORIENTED_EDGE ( 'NONE', *, *, #23380, .T. ) ;
#23431=CYLINDRICAL_SURFACE ( 'NONE', #2, 145.0000000000000284 ) ;
#23434=EDGE_CURVE ( 'NONE', #18342, #5818, #10389, .T. ) ;
#23455=EDGE_LOOP ( 'NONE', ( #19451, #23168, #2155, #20127 ) ) ;
#23466=ORIENTED_EDGE ( 'NONE', *, *, #8841, .T. ) ;
#23469=DIRECTION ( 'NONE',  ( -0.000000000000000000, 0.000000000000000000, 1.000000000000000000 ) ) ;
#23477=CIRCLE ( 'NONE', #16170, 145.0000000000000284 ) ;
#23497=CIRCLE ( 'NONE', #22328, 145.0000000000000284 ) ;
#23504=CIRCLE ( 'NONE', #15017, 7.500000000000000888 ) ;
#23510=ORIENTED_EDGE ( 'NONE', *, *, #21284, .T. ) ;
#23516=PLANE ( 'NONE',  #1498 ) ;
#23522=CARTESIAN_POINT ( 'NONE',  ( -137.5000000000000000, -5.062647941322544249E-13, -90.00000000000000000 ) ) ;
#23531=EDGE_CURVE ( 'NONE', #21395, #4516, #22331, .T. ) ;
#23533=VERTEX_POINT ( 'NONE', #2361 ) ;
#23539=DIRECTION ( 'NONE',  ( 1.000000000000000000, 0.000000000000000000, 0.000000000000000000 ) ) ;
#23567=CARTESIAN_POINT ( 'NONE',  ( 79.04925354955338435, -121.5574576620390843, 90.00000000000000000 ) ) ;
#23568=DIRECTION ( 'NONE',  ( 0.000000000000000000, 0.000000000000000000, 1.000000000000000000 ) ) ;
#23585=DIRECTION ( 'NONE',  ( 0.000000000000000000, 0.000000000000000000, 1.000000000000000000 ) ) ;
#23592=ORIENTED_EDGE ( 'NONE', *, *, #10970, .F. ) ;
#23597=DIRECTION ( 'NONE',  ( -0.000000000000000000, -0.000000000000000000, 1.000000000000000000 ) ) ;
#23598=CYLINDRICAL_SURFACE ( 'NONE', #10031, 145.0000000000000284 ) ;
#23599=ORIENTED_EDGE ( 'NONE', *, *, #10844, .F. ) ;
#23602=ORIENTED_EDGE ( 'NONE', *, *, #9791, .F. ) ;
#23612=CYLINDRICAL_SURFACE ( 'NONE', #19656, 145.0000000000000284 ) ;
#23625=FACE_OUTER_BOUND ( 'NONE', #11606, .T. ) ;
#23638=CARTESIAN_POINT ( 'NONE',  ( 0.000000000000000000, 0.000000000000000000, -90.00000000000000000 ) ) ;
#23645=CARTESIAN_POINT ( 'NONE',  ( -44.80746418436748968, 137.9031948627972781, -90.00000000000000000 ) ) ;
#23654=DIRECTION ( 'NONE',  ( 1.000000000000000000, 0.000000000000000000, -0.000000000000000000 ) ) ;
#23663=DIRECTION ( 'NONE',  ( -0.000000000000000000, -0.000000000000000000, 1.000000000000000000 ) ) ;
#23669=ORIENTED_EDGE ( 'NONE', *, *, #9577, .T. ) ;
#23674=EDGE_CURVE ( 'NONE', #6206, #19753, #2285, .T. ) ;
#23677=CARTESIAN_POINT ( 'NONE',  ( -117.3074641843675749, 85.22886158240835641, -90.00000000000000000 ) ) ;
#23680=ORIENTED_EDGE ( 'NONE', *, *, #18706, .T. ) ;
#23722=DIRECTION ( 'NONE',  ( 1.000000000000000000, 0.000000000000000000, 0.000000000000000000 ) ) ;
#23743=EDGE_LOOP ( 'NONE', ( #17143, #23592, #8036, #4631 ) ) ;
#23744=EDGE_CURVE ( 'NONE', #11081, #13199, #1518, .T. ) ;
#23751=ADVANCED_FACE ( 'NONE', ( #1263 ), #23598, .T. ) ;
#23752=ORIENTED_EDGE ( 'NONE', *, *, #14592, .T. ) ;
#23753=CARTESIAN_POINT ( 'NONE',  ( 117.3074641843682144, -85.22886158240748955, 90.00000000000000000 ) ) ;
#23758=CARTESIAN_POINT ( 'NONE',  ( -37.30746418436648071, -137.9031948627975908, -90.00000000000000000 ) ) ;
#23769=CIRCLE ( 'NONE', #12637, 145.0000000000000284 ) ;
#23773=AXIS2_PLACEMENT_3D ( 'NONE', #18485, #6948, #5023 ) ;
#23788=CIRCLE ( 'NONE', #9944, 145.0000000000000284 ) ;
#23789=DIRECTION ( 'NONE',  ( 1.000000000000000000, 0.000000000000000000, 0.000000000000000000 ) ) ;
#23796=ORIENTED_EDGE ( 'NONE', *, *, #1951, .F. ) ;
#23907=COLOUR_RGB('Sky Blue',0.24,0.69,0.87);
#23908=FILL_AREA_STYLE_COLOUR('',#23907);
#23909=FILL_AREA_STYLE('',(#23908));
#23910=SURFACE_STYLE_FILL_AREA(#23909);
#23911=SURFACE_SIDE_STYLE('',(#23910));
#23912=SURFACE_STYLE_USAGE(.BOTH.,#23911);
#23913=PRESENTATION_STYLE_ASSIGNMENT((#23912));
ENDSEC;
END-ISO-10303-21;
